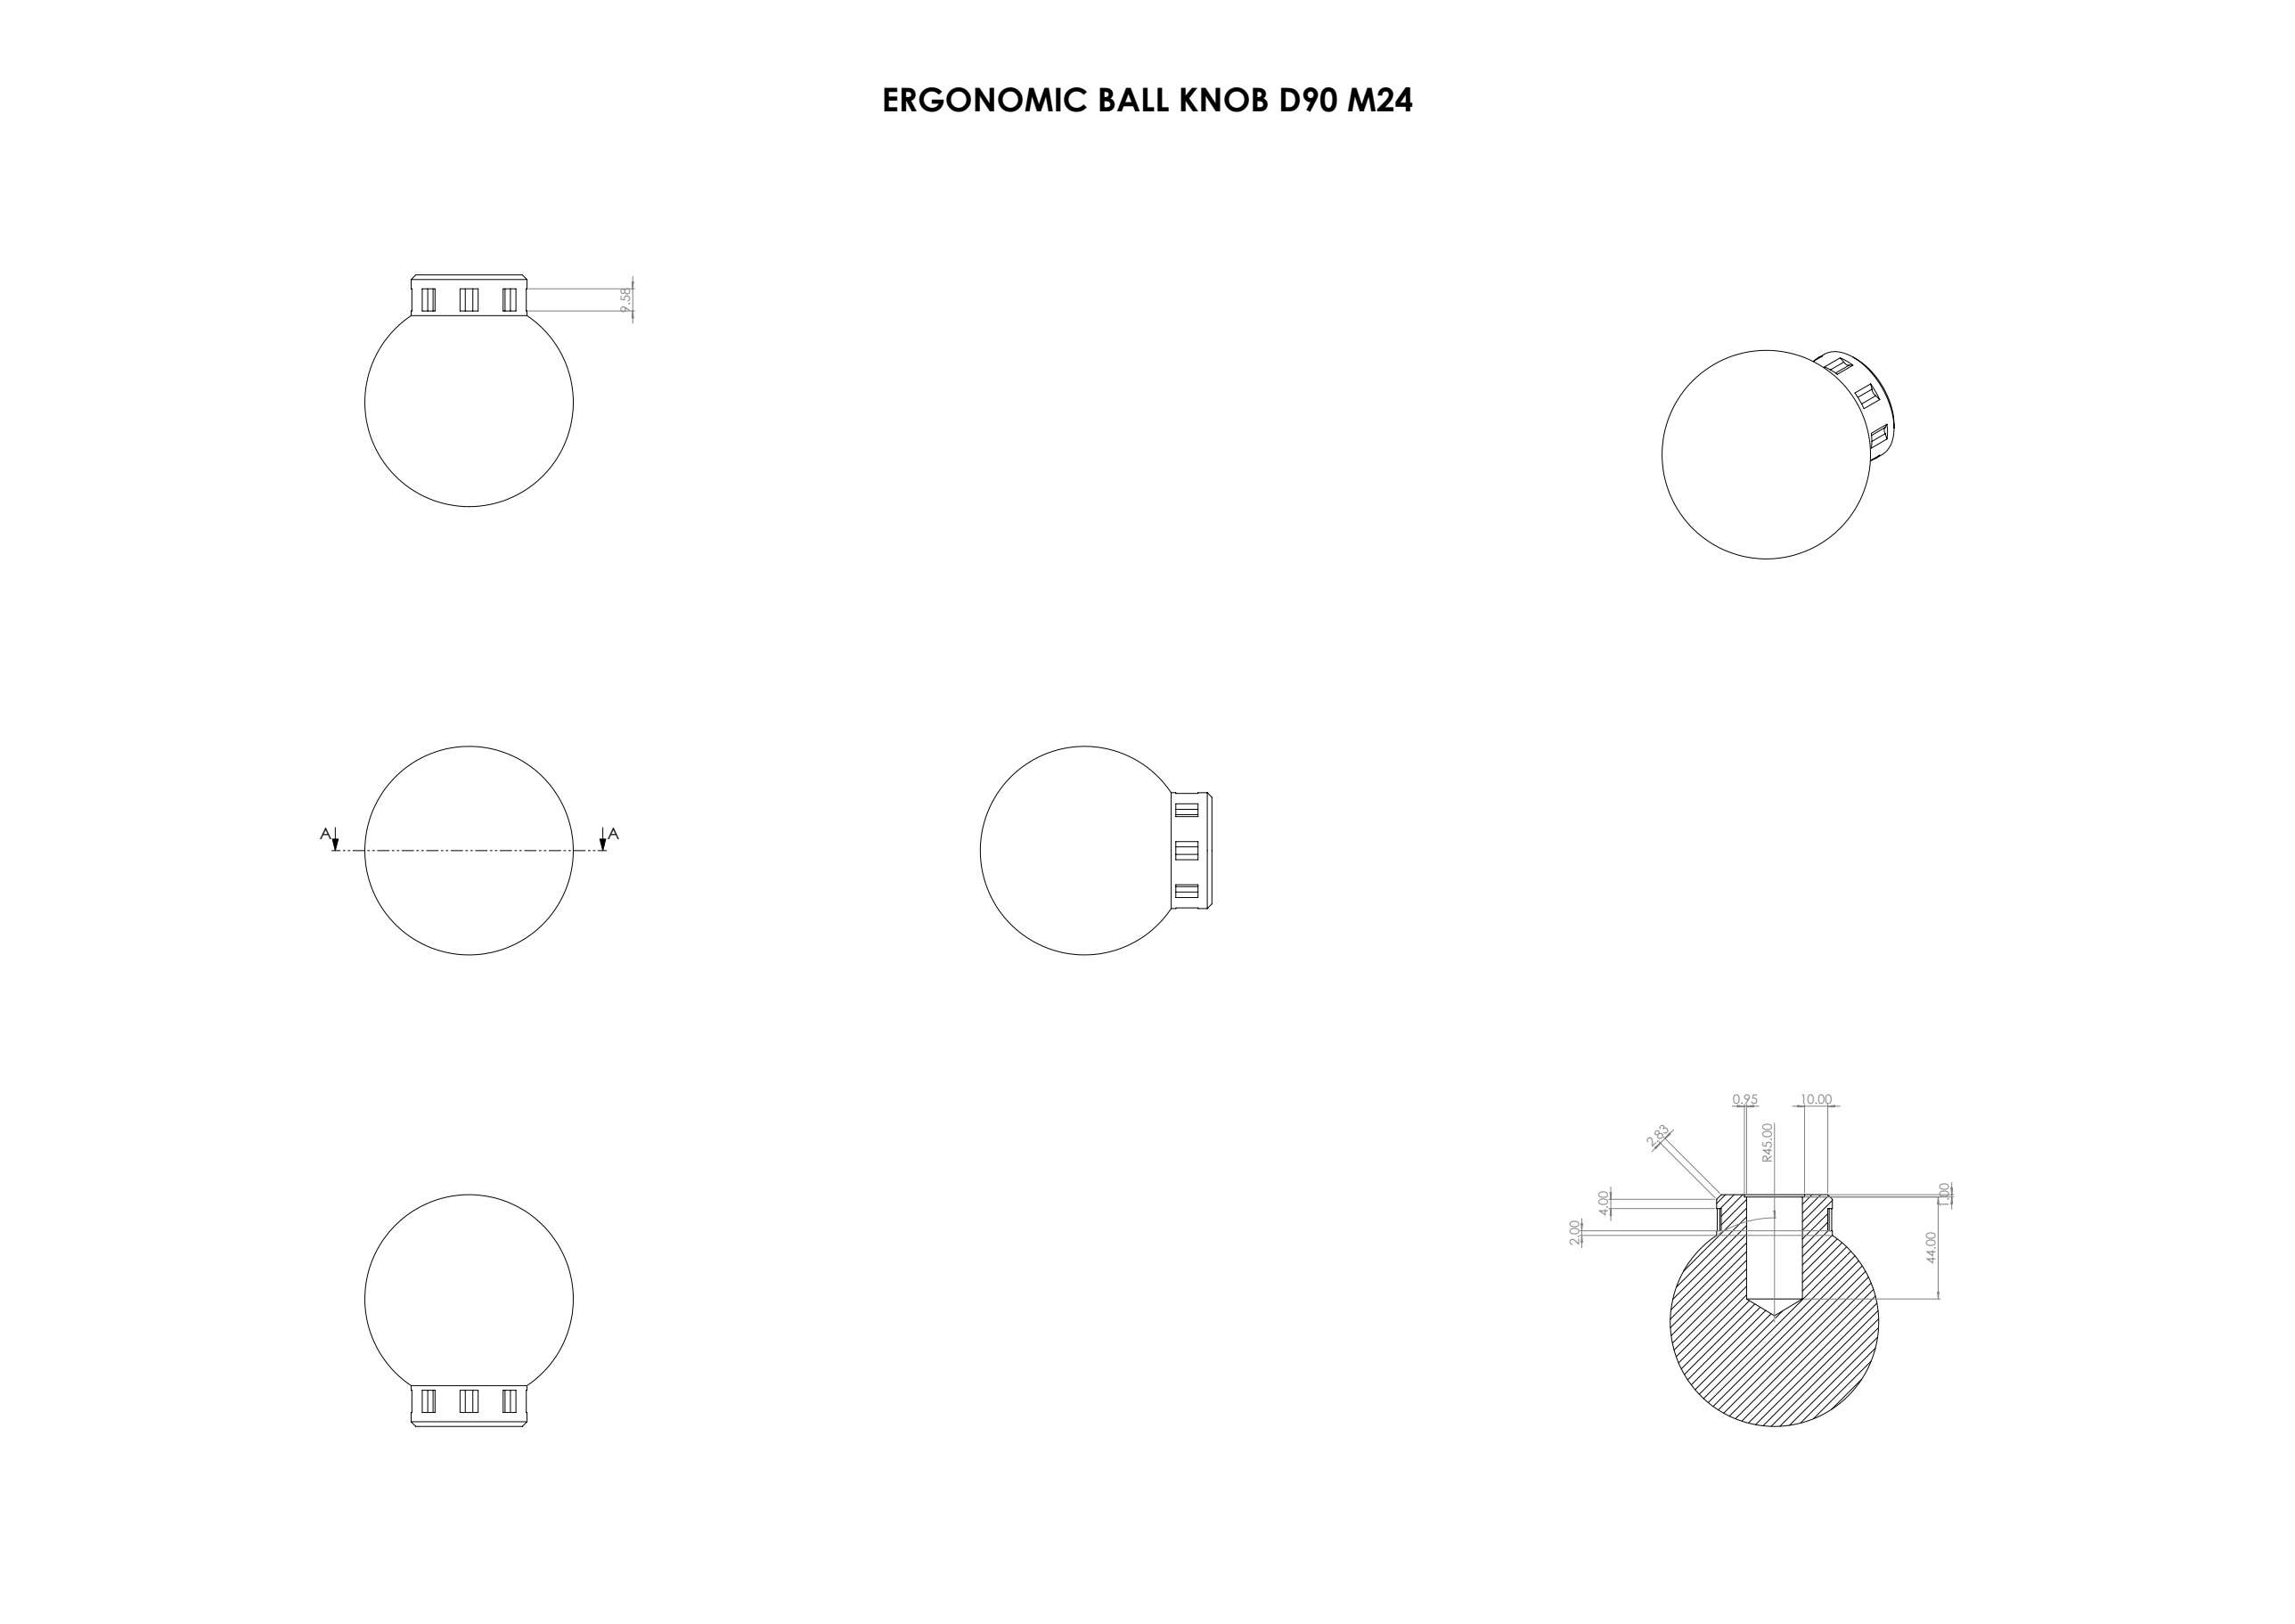
ISO-10303-21;
HEADER;
/* Generated by software containing ST-Developer
 * from STEP Tools, Inc. (www.steptools.com) 
 */

FILE_DESCRIPTION(
/* description */ (''),
/* implementation_level */ '2;1');

FILE_NAME(
/* name */ '06_Ergonomic_Ball_Knob_D90_M24.step',
/* time_stamp */ '2026-10-19T23:58:09-07:00',
/* author */ (''),
/* organization */ (''),
/* preprocessor_version */ 'ST-DEVELOPER v20.2',
/* originating_system */ 'Autodesk Translation Framework v15.15.0.0',
/* authorisation */ '');

FILE_SCHEMA (('AP203_CONFIGURATION_CONTROLLED_3D_DESIGN_OF_MECHANICAL_PARTS_AND_ASSEMBLIES_MIM_LF { 1 0 10303 203 3 1 4 }',
'AUTOMOTIVE_DESIGN { 1 0 10303 214 3 1 1 }','INTEGRATED_CNC_SCHEMA','MODEL_BASED_INTEGRATED_MANUFACTURING_SCHEMA',
'PROCESS_PLANNING_SCHEMA','AP242_MANAGED_MODEL_BASED_3D_ENGINEERING_MIM_LF { 1 0 10303 442 3 1 4 }'));
ENDSEC;

DATA;
#10=MECHANICAL_DESIGN_GEOMETRIC_PRESENTATION_REPRESENTATION('',(#419),#70757);
#135=SPHERICAL_SURFACE('',#28394,4.5);
#389=SHAPE_REPRESENTATION_RELATIONSHIP('SRR','None',#70830,#404);
#404=ADVANCED_BREP_SHAPE_REPRESENTATION('',(#479),#70754);
#419=STYLED_ITEM('',(#71040),#479);
#479=MANIFOLD_SOLID_BREP('Knob',#26884);
#730=CYLINDRICAL_SURFACE('',#28307,0.25);
#731=CYLINDRICAL_SURFACE('',#28312,0.25);
#732=CYLINDRICAL_SURFACE('',#28317,0.25);
#733=CYLINDRICAL_SURFACE('',#28322,0.25);
#734=CYLINDRICAL_SURFACE('',#28327,0.25);
#735=CYLINDRICAL_SURFACE('',#28332,0.25);
#736=CYLINDRICAL_SURFACE('',#28337,0.25);
#737=CYLINDRICAL_SURFACE('',#28342,0.25);
#738=CYLINDRICAL_SURFACE('',#28380,1.3);
#739=CYLINDRICAL_SURFACE('',#28385,1.205);
#740=CYLINDRICAL_SURFACE('',#28392,2.5);
#878=FACE_BOUND('',#5169,.T.);
#879=FACE_BOUND('',#5173,.T.);
#880=FACE_BOUND('',#5176,.T.);
#881=FACE_BOUND('',#5177,.T.);
#882=FACE_BOUND('',#5178,.T.);
#883=FACE_BOUND('',#5179,.T.);
#884=FACE_BOUND('',#5180,.T.);
#885=FACE_BOUND('',#5181,.T.);
#886=FACE_BOUND('',#5182,.T.);
#2392=PLANE('',#28306);
#2393=PLANE('',#28310);
#2394=PLANE('',#28311);
#2395=PLANE('',#28315);
#2396=PLANE('',#28316);
#2397=PLANE('',#28320);
#2398=PLANE('',#28321);
#2399=PLANE('',#28325);
#2400=PLANE('',#28326);
#2401=PLANE('',#28330);
#2402=PLANE('',#28331);
#2403=PLANE('',#28335);
#2404=PLANE('',#28336);
#2405=PLANE('',#28340);
#2406=PLANE('',#28341);
#2407=PLANE('',#28345);
#2408=PLANE('',#28346);
#2409=PLANE('',#28348);
#2410=PLANE('',#28350);
#2411=PLANE('',#28353);
#2412=PLANE('',#28356);
#2413=PLANE('',#28358);
#2414=PLANE('',#28360);
#2415=PLANE('',#28362);
#2416=PLANE('',#28364);
#2417=PLANE('',#28366);
#2418=PLANE('',#28368);
#2419=PLANE('',#28370);
#2420=PLANE('',#28372);
#2421=PLANE('',#28374);
#2422=PLANE('',#28376);
#2423=PLANE('',#28378);
#2424=PLANE('',#28383);
#2425=PLANE('',#28388);
#3605=FACE_OUTER_BOUND('',#5127,.T.);
#3606=FACE_OUTER_BOUND('',#5128,.T.);
#3607=FACE_OUTER_BOUND('',#5129,.T.);
#3608=FACE_OUTER_BOUND('',#5130,.T.);
#3609=FACE_OUTER_BOUND('',#5131,.T.);
#3610=FACE_OUTER_BOUND('',#5132,.T.);
#3611=FACE_OUTER_BOUND('',#5133,.T.);
#3612=FACE_OUTER_BOUND('',#5134,.T.);
#3613=FACE_OUTER_BOUND('',#5135,.T.);
#3614=FACE_OUTER_BOUND('',#5136,.T.);
#3615=FACE_OUTER_BOUND('',#5137,.T.);
#3616=FACE_OUTER_BOUND('',#5138,.T.);
#3617=FACE_OUTER_BOUND('',#5139,.T.);
#3618=FACE_OUTER_BOUND('',#5140,.T.);
#3619=FACE_OUTER_BOUND('',#5141,.T.);
#3620=FACE_OUTER_BOUND('',#5142,.T.);
#3621=FACE_OUTER_BOUND('',#5143,.T.);
#3622=FACE_OUTER_BOUND('',#5144,.T.);
#3623=FACE_OUTER_BOUND('',#5145,.T.);
#3624=FACE_OUTER_BOUND('',#5146,.T.);
#3625=FACE_OUTER_BOUND('',#5147,.T.);
#3626=FACE_OUTER_BOUND('',#5148,.T.);
#3627=FACE_OUTER_BOUND('',#5149,.T.);
#3628=FACE_OUTER_BOUND('',#5150,.T.);
#3629=FACE_OUTER_BOUND('',#5151,.T.);
#3630=FACE_OUTER_BOUND('',#5152,.T.);
#3631=FACE_OUTER_BOUND('',#5153,.T.);
#3632=FACE_OUTER_BOUND('',#5154,.T.);
#3633=FACE_OUTER_BOUND('',#5155,.T.);
#3634=FACE_OUTER_BOUND('',#5156,.T.);
#3635=FACE_OUTER_BOUND('',#5157,.T.);
#3636=FACE_OUTER_BOUND('',#5158,.T.);
#3637=FACE_OUTER_BOUND('',#5159,.T.);
#3638=FACE_OUTER_BOUND('',#5160,.T.);
#3639=FACE_OUTER_BOUND('',#5161,.T.);
#3640=FACE_OUTER_BOUND('',#5162,.T.);
#3641=FACE_OUTER_BOUND('',#5163,.T.);
#3642=FACE_OUTER_BOUND('',#5164,.T.);
#3643=FACE_OUTER_BOUND('',#5165,.T.);
#3644=FACE_OUTER_BOUND('',#5166,.T.);
#3645=FACE_OUTER_BOUND('',#5167,.T.);
#3646=FACE_OUTER_BOUND('',#5168,.T.);
#3647=FACE_OUTER_BOUND('',#5170,.T.);
#3648=FACE_OUTER_BOUND('',#5171,.T.);
#3649=FACE_OUTER_BOUND('',#5172,.T.);
#3650=FACE_OUTER_BOUND('',#5174,.T.);
#3651=FACE_OUTER_BOUND('',#5175,.T.);
#3652=FACE_OUTER_BOUND('',#5183,.T.);
#5127=EDGE_LOOP('',(#22944,#22945,#22946,#22947));
#5128=EDGE_LOOP('',(#22948,#22949,#22950,#22951));
#5129=EDGE_LOOP('',(#22952,#22953,#22954,#22955));
#5130=EDGE_LOOP('',(#22956,#22957,#22958,#22959));
#5131=EDGE_LOOP('',(#22960,#22961,#22962,#22963));
#5132=EDGE_LOOP('',(#22964,#22965,#22966,#22967));
#5133=EDGE_LOOP('',(#22968,#22969,#22970,#22971));
#5134=EDGE_LOOP('',(#22972,#22973,#22974,#22975));
#5135=EDGE_LOOP('',(#22976,#22977,#22978,#22979));
#5136=EDGE_LOOP('',(#22980,#22981,#22982,#22983));
#5137=EDGE_LOOP('',(#22984,#22985,#22986,#22987));
#5138=EDGE_LOOP('',(#22988,#22989,#22990,#22991));
#5139=EDGE_LOOP('',(#22992,#22993,#22994,#22995));
#5140=EDGE_LOOP('',(#22996,#22997,#22998,#22999));
#5141=EDGE_LOOP('',(#23000,#23001,#23002,#23003));
#5142=EDGE_LOOP('',(#23004,#23005,#23006,#23007));
#5143=EDGE_LOOP('',(#23008,#23009,#23010,#23011));
#5144=EDGE_LOOP('',(#23012,#23013,#23014,#23015));
#5145=EDGE_LOOP('',(#23016,#23017,#23018,#23019));
#5146=EDGE_LOOP('',(#23020,#23021,#23022,#23023));
#5147=EDGE_LOOP('',(#23024,#23025,#23026,#23027));
#5148=EDGE_LOOP('',(#23028,#23029,#23030,#23031));
#5149=EDGE_LOOP('',(#23032,#23033,#23034,#23035));
#5150=EDGE_LOOP('',(#23036,#23037,#23038,#23039));
#5151=EDGE_LOOP('',(#23040,#23041,#23042,#23043));
#5152=EDGE_LOOP('',(#23044,#23045,#23046,#23047));
#5153=EDGE_LOOP('',(#23048,#23049,#23050,#23051,#23052));
#5154=EDGE_LOOP('',(#23053,#23054,#23055,#23056,#23057));
#5155=EDGE_LOOP('',(#23058,#23059,#23060,#23061));
#5156=EDGE_LOOP('',(#23062,#23063,#23064,#23065));
#5157=EDGE_LOOP('',(#23066,#23067,#23068,#23069));
#5158=EDGE_LOOP('',(#23070,#23071,#23072,#23073));
#5159=EDGE_LOOP('',(#23074,#23075,#23076,#23077));
#5160=EDGE_LOOP('',(#23078,#23079,#23080,#23081));
#5161=EDGE_LOOP('',(#23082,#23083,#23084,#23085));
#5162=EDGE_LOOP('',(#23086,#23087,#23088,#23089));
#5163=EDGE_LOOP('',(#23090,#23091,#23092,#23093));
#5164=EDGE_LOOP('',(#23094,#23095,#23096,#23097));
#5165=EDGE_LOOP('',(#23098,#23099,#23100,#23101));
#5166=EDGE_LOOP('',(#23102,#23103,#23104,#23105));
#5167=EDGE_LOOP('',(#23106,#23107,#23108,#23109));
#5168=EDGE_LOOP('',(#23110));
#5169=EDGE_LOOP('',(#23111));
#5170=EDGE_LOOP('',(#23112,#23113,#23114,#23115));
#5171=EDGE_LOOP('',(#23116,#23117,#23118));
#5172=EDGE_LOOP('',(#23119));
#5173=EDGE_LOOP('',(#23120));
#5174=EDGE_LOOP('',(#23121,#23122,#23123,#23124));
#5175=EDGE_LOOP('',(#23125,#23126,#23127,#23128,#23129,#23130,#23131,#23132,
#23133,#23134,#23135,#23136));
#5176=EDGE_LOOP('',(#23137,#23138,#23139,#23140));
#5177=EDGE_LOOP('',(#23141,#23142,#23143,#23144));
#5178=EDGE_LOOP('',(#23145,#23146,#23147,#23148));
#5179=EDGE_LOOP('',(#23149,#23150,#23151,#23152));
#5180=EDGE_LOOP('',(#23153,#23154,#23155,#23156));
#5181=EDGE_LOOP('',(#23157,#23158,#23159,#23160));
#5182=EDGE_LOOP('',(#23161,#23162,#23163,#23164));
#5183=EDGE_LOOP('',(#23165,#23166,#23167));
#7543=LINE('',#63698,#10040);
#7544=LINE('',#63700,#10041);
#7545=LINE('',#63702,#10042);
#7546=LINE('',#63703,#10043);
#7547=LINE('',#63708,#10044);
#7548=LINE('',#63712,#10045);
#7549=LINE('',#63714,#10046);
#7550=LINE('',#63715,#10047);
#7551=LINE('',#63719,#10048);
#7552=LINE('',#63721,#10049);
#7553=LINE('',#63723,#10050);
#7554=LINE('',#63724,#10051);
#7555=LINE('',#63729,#10052);
#7556=LINE('',#63733,#10053);
#7557=LINE('',#63735,#10054);
#7558=LINE('',#63736,#10055);
#7559=LINE('',#63740,#10056);
#7560=LINE('',#63742,#10057);
#7561=LINE('',#63744,#10058);
#7562=LINE('',#63745,#10059);
#7563=LINE('',#63750,#10060);
#7564=LINE('',#63754,#10061);
#7565=LINE('',#63756,#10062);
#7566=LINE('',#63757,#10063);
#7567=LINE('',#63761,#10064);
#7568=LINE('',#63763,#10065);
#7569=LINE('',#63765,#10066);
#7570=LINE('',#63766,#10067);
#7571=LINE('',#63771,#10068);
#7572=LINE('',#63775,#10069);
#7573=LINE('',#63777,#10070);
#7574=LINE('',#63778,#10071);
#7575=LINE('',#63782,#10072);
#7576=LINE('',#63784,#10073);
#7577=LINE('',#63786,#10074);
#7578=LINE('',#63787,#10075);
#7579=LINE('',#63792,#10076);
#7580=LINE('',#63796,#10077);
#7581=LINE('',#63798,#10078);
#7582=LINE('',#63799,#10079);
#7583=LINE('',#63803,#10080);
#7584=LINE('',#63805,#10081);
#7585=LINE('',#63807,#10082);
#7586=LINE('',#63808,#10083);
#7587=LINE('',#63813,#10084);
#7588=LINE('',#63817,#10085);
#7589=LINE('',#63819,#10086);
#7590=LINE('',#63820,#10087);
#7591=LINE('',#63824,#10088);
#7592=LINE('',#63826,#10089);
#7593=LINE('',#63828,#10090);
#7594=LINE('',#63829,#10091);
#7595=LINE('',#63834,#10092);
#7596=LINE('',#63838,#10093);
#7597=LINE('',#63840,#10094);
#7598=LINE('',#63841,#10095);
#7599=LINE('',#63845,#10096);
#7600=LINE('',#63847,#10097);
#7601=LINE('',#63849,#10098);
#7602=LINE('',#63850,#10099);
#7603=LINE('',#63855,#10100);
#7604=LINE('',#63859,#10101);
#7605=LINE('',#63861,#10102);
#7606=LINE('',#63862,#10103);
#7607=LINE('',#63903,#10104);
#7608=LINE('',#63910,#10105);
#7609=LINE('',#63914,#10106);
#7610=LINE('',#63921,#10107);
#7611=LINE('',#63925,#10108);
#7612=LINE('',#63926,#10109);
#10040=VECTOR('',#33406,1.);
#10041=VECTOR('',#33407,1.);
#10042=VECTOR('',#33408,1.);
#10043=VECTOR('',#33409,1.);
#10044=VECTOR('',#33414,1.);
#10045=VECTOR('',#33419,1.);
#10046=VECTOR('',#33420,1.);
#10047=VECTOR('',#33421,1.);
#10048=VECTOR('',#33424,1.);
#10049=VECTOR('',#33425,1.);
#10050=VECTOR('',#33426,1.);
#10051=VECTOR('',#33427,1.);
#10052=VECTOR('',#33432,1.);
#10053=VECTOR('',#33437,1.);
#10054=VECTOR('',#33438,1.);
#10055=VECTOR('',#33439,1.);
#10056=VECTOR('',#33442,1.);
#10057=VECTOR('',#33443,1.);
#10058=VECTOR('',#33444,1.);
#10059=VECTOR('',#33445,1.);
#10060=VECTOR('',#33450,1.);
#10061=VECTOR('',#33455,1.);
#10062=VECTOR('',#33456,1.);
#10063=VECTOR('',#33457,1.);
#10064=VECTOR('',#33460,1.);
#10065=VECTOR('',#33461,1.);
#10066=VECTOR('',#33462,1.);
#10067=VECTOR('',#33463,1.);
#10068=VECTOR('',#33468,1.);
#10069=VECTOR('',#33473,1.);
#10070=VECTOR('',#33474,1.);
#10071=VECTOR('',#33475,1.);
#10072=VECTOR('',#33478,1.);
#10073=VECTOR('',#33479,1.);
#10074=VECTOR('',#33480,1.);
#10075=VECTOR('',#33481,1.);
#10076=VECTOR('',#33486,1.);
#10077=VECTOR('',#33491,1.);
#10078=VECTOR('',#33492,1.);
#10079=VECTOR('',#33493,1.);
#10080=VECTOR('',#33496,1.);
#10081=VECTOR('',#33497,1.);
#10082=VECTOR('',#33498,1.);
#10083=VECTOR('',#33499,1.);
#10084=VECTOR('',#33504,1.);
#10085=VECTOR('',#33509,1.);
#10086=VECTOR('',#33510,1.);
#10087=VECTOR('',#33511,1.);
#10088=VECTOR('',#33514,1.);
#10089=VECTOR('',#33515,1.);
#10090=VECTOR('',#33516,1.);
#10091=VECTOR('',#33517,1.);
#10092=VECTOR('',#33522,1.);
#10093=VECTOR('',#33527,1.);
#10094=VECTOR('',#33528,1.);
#10095=VECTOR('',#33529,1.);
#10096=VECTOR('',#33532,1.);
#10097=VECTOR('',#33533,1.);
#10098=VECTOR('',#33534,1.);
#10099=VECTOR('',#33535,1.);
#10100=VECTOR('',#33540,1.);
#10101=VECTOR('',#33545,1.);
#10102=VECTOR('',#33546,1.);
#10103=VECTOR('',#33547,1.);
#10104=VECTOR('',#33620,1.3);
#10105=VECTOR('',#33629,1.205);
#10106=VECTOR('',#33634,1.205);
#10107=VECTOR('',#33643,2.4);
#10108=VECTOR('',#33648,2.5);
#10109=VECTOR('',#33649,2.5);
#10881=CIRCLE('',#28308,0.25);
#10882=CIRCLE('',#28309,0.25);
#10883=CIRCLE('',#28313,0.25);
#10884=CIRCLE('',#28314,0.25);
#10885=CIRCLE('',#28318,0.25);
#10886=CIRCLE('',#28319,0.25);
#10887=CIRCLE('',#28323,0.25);
#10888=CIRCLE('',#28324,0.25);
#10889=CIRCLE('',#28328,0.25);
#10890=CIRCLE('',#28329,0.25);
#10891=CIRCLE('',#28333,0.25);
#10892=CIRCLE('',#28334,0.25);
#10893=CIRCLE('',#28338,0.25);
#10894=CIRCLE('',#28339,0.25);
#10895=CIRCLE('',#28343,0.25);
#10896=CIRCLE('',#28344,0.25);
#10897=CIRCLE('',#28347,2.5);
#10898=CIRCLE('',#28349,2.5);
#10899=CIRCLE('',#28351,2.5);
#10900=CIRCLE('',#28352,2.5);
#10901=CIRCLE('',#28354,2.5);
#10902=CIRCLE('',#28355,2.5);
#10903=CIRCLE('',#28357,2.5);
#10904=CIRCLE('',#28359,2.5);
#10905=CIRCLE('',#28361,2.5);
#10906=CIRCLE('',#28363,2.5);
#10907=CIRCLE('',#28365,2.5);
#10908=CIRCLE('',#28367,2.5);
#10909=CIRCLE('',#28369,2.5);
#10910=CIRCLE('',#28371,2.5);
#10911=CIRCLE('',#28373,2.5);
#10912=CIRCLE('',#28375,2.5);
#10913=CIRCLE('',#28377,2.5);
#10914=CIRCLE('',#28379,2.5);
#10915=CIRCLE('',#28381,1.3);
#10916=CIRCLE('',#28382,1.3);
#10917=CIRCLE('',#28384,1.205);
#10918=CIRCLE('',#28386,1.205);
#10919=CIRCLE('',#28389,2.3);
#10920=CIRCLE('',#28391,2.5);
#10921=CIRCLE('',#28393,2.5);
#10922=CIRCLE('',#28395,4.5);
#12856=VERTEX_POINT('',#63696);
#12857=VERTEX_POINT('',#63697);
#12858=VERTEX_POINT('',#63699);
#12859=VERTEX_POINT('',#63701);
#12860=VERTEX_POINT('',#63705);
#12861=VERTEX_POINT('',#63707);
#12862=VERTEX_POINT('',#63711);
#12863=VERTEX_POINT('',#63713);
#12864=VERTEX_POINT('',#63717);
#12865=VERTEX_POINT('',#63718);
#12866=VERTEX_POINT('',#63720);
#12867=VERTEX_POINT('',#63722);
#12868=VERTEX_POINT('',#63726);
#12869=VERTEX_POINT('',#63728);
#12870=VERTEX_POINT('',#63732);
#12871=VERTEX_POINT('',#63734);
#12872=VERTEX_POINT('',#63738);
#12873=VERTEX_POINT('',#63739);
#12874=VERTEX_POINT('',#63741);
#12875=VERTEX_POINT('',#63743);
#12876=VERTEX_POINT('',#63747);
#12877=VERTEX_POINT('',#63749);
#12878=VERTEX_POINT('',#63753);
#12879=VERTEX_POINT('',#63755);
#12880=VERTEX_POINT('',#63759);
#12881=VERTEX_POINT('',#63760);
#12882=VERTEX_POINT('',#63762);
#12883=VERTEX_POINT('',#63764);
#12884=VERTEX_POINT('',#63768);
#12885=VERTEX_POINT('',#63770);
#12886=VERTEX_POINT('',#63774);
#12887=VERTEX_POINT('',#63776);
#12888=VERTEX_POINT('',#63780);
#12889=VERTEX_POINT('',#63781);
#12890=VERTEX_POINT('',#63783);
#12891=VERTEX_POINT('',#63785);
#12892=VERTEX_POINT('',#63789);
#12893=VERTEX_POINT('',#63791);
#12894=VERTEX_POINT('',#63795);
#12895=VERTEX_POINT('',#63797);
#12896=VERTEX_POINT('',#63801);
#12897=VERTEX_POINT('',#63802);
#12898=VERTEX_POINT('',#63804);
#12899=VERTEX_POINT('',#63806);
#12900=VERTEX_POINT('',#63810);
#12901=VERTEX_POINT('',#63812);
#12902=VERTEX_POINT('',#63816);
#12903=VERTEX_POINT('',#63818);
#12904=VERTEX_POINT('',#63822);
#12905=VERTEX_POINT('',#63823);
#12906=VERTEX_POINT('',#63825);
#12907=VERTEX_POINT('',#63827);
#12908=VERTEX_POINT('',#63831);
#12909=VERTEX_POINT('',#63833);
#12910=VERTEX_POINT('',#63837);
#12911=VERTEX_POINT('',#63839);
#12912=VERTEX_POINT('',#63843);
#12913=VERTEX_POINT('',#63844);
#12914=VERTEX_POINT('',#63846);
#12915=VERTEX_POINT('',#63848);
#12916=VERTEX_POINT('',#63852);
#12917=VERTEX_POINT('',#63854);
#12918=VERTEX_POINT('',#63858);
#12919=VERTEX_POINT('',#63860);
#12920=VERTEX_POINT('',#63868);
#12921=VERTEX_POINT('',#63872);
#12922=VERTEX_POINT('',#63900);
#12923=VERTEX_POINT('',#63902);
#12924=VERTEX_POINT('',#63906);
#12925=VERTEX_POINT('',#63909);
#12926=VERTEX_POINT('',#63913);
#12927=VERTEX_POINT('',#63916);
#12928=VERTEX_POINT('',#63919);
#12929=VERTEX_POINT('',#63923);
#12930=VERTEX_POINT('',#63928);
#16325=EDGE_CURVE('',#12856,#12857,#7543,.F.);
#16326=EDGE_CURVE('',#12857,#12858,#7544,.T.);
#16327=EDGE_CURVE('',#12858,#12859,#7545,.F.);
#16328=EDGE_CURVE('',#12859,#12856,#7546,.T.);
#16329=EDGE_CURVE('',#12860,#12857,#10881,.T.);
#16330=EDGE_CURVE('',#12861,#12860,#7547,.T.);
#16331=EDGE_CURVE('',#12861,#12858,#10882,.T.);
#16332=EDGE_CURVE('',#12862,#12861,#7548,.F.);
#16333=EDGE_CURVE('',#12860,#12863,#7549,.F.);
#16334=EDGE_CURVE('',#12863,#12862,#7550,.T.);
#16335=EDGE_CURVE('',#12864,#12865,#7551,.F.);
#16336=EDGE_CURVE('',#12865,#12866,#7552,.T.);
#16337=EDGE_CURVE('',#12866,#12867,#7553,.F.);
#16338=EDGE_CURVE('',#12867,#12864,#7554,.T.);
#16339=EDGE_CURVE('',#12865,#12868,#10883,.T.);
#16340=EDGE_CURVE('',#12869,#12868,#7555,.T.);
#16341=EDGE_CURVE('',#12866,#12869,#10884,.T.);
#16342=EDGE_CURVE('',#12870,#12869,#7556,.F.);
#16343=EDGE_CURVE('',#12868,#12871,#7557,.F.);
#16344=EDGE_CURVE('',#12871,#12870,#7558,.T.);
#16345=EDGE_CURVE('',#12872,#12873,#7559,.F.);
#16346=EDGE_CURVE('',#12873,#12874,#7560,.T.);
#16347=EDGE_CURVE('',#12874,#12875,#7561,.F.);
#16348=EDGE_CURVE('',#12875,#12872,#7562,.T.);
#16349=EDGE_CURVE('',#12876,#12873,#10885,.T.);
#16350=EDGE_CURVE('',#12877,#12876,#7563,.T.);
#16351=EDGE_CURVE('',#12877,#12874,#10886,.T.);
#16352=EDGE_CURVE('',#12878,#12877,#7564,.F.);
#16353=EDGE_CURVE('',#12876,#12879,#7565,.F.);
#16354=EDGE_CURVE('',#12879,#12878,#7566,.T.);
#16355=EDGE_CURVE('',#12880,#12881,#7567,.F.);
#16356=EDGE_CURVE('',#12881,#12882,#7568,.T.);
#16357=EDGE_CURVE('',#12882,#12883,#7569,.F.);
#16358=EDGE_CURVE('',#12883,#12880,#7570,.T.);
#16359=EDGE_CURVE('',#12881,#12884,#10887,.T.);
#16360=EDGE_CURVE('',#12885,#12884,#7571,.T.);
#16361=EDGE_CURVE('',#12882,#12885,#10888,.T.);
#16362=EDGE_CURVE('',#12886,#12885,#7572,.F.);
#16363=EDGE_CURVE('',#12884,#12887,#7573,.F.);
#16364=EDGE_CURVE('',#12887,#12886,#7574,.T.);
#16365=EDGE_CURVE('',#12888,#12889,#7575,.F.);
#16366=EDGE_CURVE('',#12889,#12890,#7576,.T.);
#16367=EDGE_CURVE('',#12890,#12891,#7577,.F.);
#16368=EDGE_CURVE('',#12891,#12888,#7578,.T.);
#16369=EDGE_CURVE('',#12892,#12889,#10889,.T.);
#16370=EDGE_CURVE('',#12893,#12892,#7579,.T.);
#16371=EDGE_CURVE('',#12893,#12890,#10890,.T.);
#16372=EDGE_CURVE('',#12894,#12893,#7580,.F.);
#16373=EDGE_CURVE('',#12892,#12895,#7581,.F.);
#16374=EDGE_CURVE('',#12895,#12894,#7582,.T.);
#16375=EDGE_CURVE('',#12896,#12897,#7583,.F.);
#16376=EDGE_CURVE('',#12897,#12898,#7584,.T.);
#16377=EDGE_CURVE('',#12898,#12899,#7585,.F.);
#16378=EDGE_CURVE('',#12899,#12896,#7586,.T.);
#16379=EDGE_CURVE('',#12897,#12900,#10891,.T.);
#16380=EDGE_CURVE('',#12901,#12900,#7587,.T.);
#16381=EDGE_CURVE('',#12898,#12901,#10892,.T.);
#16382=EDGE_CURVE('',#12902,#12901,#7588,.F.);
#16383=EDGE_CURVE('',#12900,#12903,#7589,.F.);
#16384=EDGE_CURVE('',#12903,#12902,#7590,.T.);
#16385=EDGE_CURVE('',#12904,#12905,#7591,.F.);
#16386=EDGE_CURVE('',#12905,#12906,#7592,.T.);
#16387=EDGE_CURVE('',#12906,#12907,#7593,.F.);
#16388=EDGE_CURVE('',#12907,#12904,#7594,.T.);
#16389=EDGE_CURVE('',#12905,#12908,#10893,.T.);
#16390=EDGE_CURVE('',#12909,#12908,#7595,.T.);
#16391=EDGE_CURVE('',#12906,#12909,#10894,.T.);
#16392=EDGE_CURVE('',#12910,#12909,#7596,.F.);
#16393=EDGE_CURVE('',#12908,#12911,#7597,.F.);
#16394=EDGE_CURVE('',#12911,#12910,#7598,.T.);
#16395=EDGE_CURVE('',#12912,#12913,#7599,.F.);
#16396=EDGE_CURVE('',#12913,#12914,#7600,.T.);
#16397=EDGE_CURVE('',#12914,#12915,#7601,.F.);
#16398=EDGE_CURVE('',#12915,#12912,#7602,.T.);
#16399=EDGE_CURVE('',#12913,#12916,#10895,.T.);
#16400=EDGE_CURVE('',#12917,#12916,#7603,.T.);
#16401=EDGE_CURVE('',#12914,#12917,#10896,.T.);
#16402=EDGE_CURVE('',#12918,#12917,#7604,.F.);
#16403=EDGE_CURVE('',#12916,#12919,#7605,.F.);
#16404=EDGE_CURVE('',#12919,#12918,#7606,.T.);
#16405=EDGE_CURVE('',#12919,#12912,#10897,.T.);
#16406=EDGE_CURVE('',#12915,#12918,#10898,.T.);
#16407=EDGE_CURVE('',#12911,#12920,#10899,.T.);
#16408=EDGE_CURVE('',#12920,#12904,#10900,.T.);
#16409=EDGE_CURVE('',#12907,#12921,#10901,.T.);
#16410=EDGE_CURVE('',#12921,#12910,#10902,.T.);
#16411=EDGE_CURVE('',#12903,#12896,#10903,.T.);
#16412=EDGE_CURVE('',#12899,#12902,#10904,.T.);
#16413=EDGE_CURVE('',#12895,#12888,#10905,.T.);
#16414=EDGE_CURVE('',#12891,#12894,#10906,.T.);
#16415=EDGE_CURVE('',#12887,#12880,#10907,.T.);
#16416=EDGE_CURVE('',#12883,#12886,#10908,.T.);
#16417=EDGE_CURVE('',#12879,#12872,#10909,.T.);
#16418=EDGE_CURVE('',#12875,#12878,#10910,.T.);
#16419=EDGE_CURVE('',#12871,#12864,#10911,.T.);
#16420=EDGE_CURVE('',#12867,#12870,#10912,.T.);
#16421=EDGE_CURVE('',#12863,#12856,#10913,.T.);
#16422=EDGE_CURVE('',#12859,#12862,#10914,.T.);
#16423=EDGE_CURVE('',#12922,#12922,#10915,.T.);
#16424=EDGE_CURVE('',#12922,#12923,#7607,.T.);
#16425=EDGE_CURVE('',#12923,#12923,#10916,.T.);
#16426=EDGE_CURVE('',#12924,#12924,#10917,.T.);
#16427=EDGE_CURVE('',#12924,#12925,#7608,.T.);
#16428=EDGE_CURVE('',#12925,#12925,#10918,.T.);
#16429=EDGE_CURVE('',#12925,#12926,#7609,.T.);
#16430=EDGE_CURVE('',#12927,#12927,#10919,.T.);
#16431=EDGE_CURVE('',#12928,#12928,#10920,.T.);
#16432=EDGE_CURVE('',#12928,#12927,#7610,.T.);
#16433=EDGE_CURVE('',#12929,#12929,#10921,.T.);
#16434=EDGE_CURVE('',#12929,#12920,#7611,.T.);
#16435=EDGE_CURVE('',#12921,#12928,#7612,.T.);
#16436=EDGE_CURVE('',#12930,#12929,#10922,.T.);
#22944=ORIENTED_EDGE('',*,*,#16325,.T.);
#22945=ORIENTED_EDGE('',*,*,#16326,.T.);
#22946=ORIENTED_EDGE('',*,*,#16327,.T.);
#22947=ORIENTED_EDGE('',*,*,#16328,.T.);
#22948=ORIENTED_EDGE('',*,*,#16326,.F.);
#22949=ORIENTED_EDGE('',*,*,#16329,.F.);
#22950=ORIENTED_EDGE('',*,*,#16330,.F.);
#22951=ORIENTED_EDGE('',*,*,#16331,.T.);
#22952=ORIENTED_EDGE('',*,*,#16332,.T.);
#22953=ORIENTED_EDGE('',*,*,#16330,.T.);
#22954=ORIENTED_EDGE('',*,*,#16333,.T.);
#22955=ORIENTED_EDGE('',*,*,#16334,.T.);
#22956=ORIENTED_EDGE('',*,*,#16335,.T.);
#22957=ORIENTED_EDGE('',*,*,#16336,.T.);
#22958=ORIENTED_EDGE('',*,*,#16337,.T.);
#22959=ORIENTED_EDGE('',*,*,#16338,.T.);
#22960=ORIENTED_EDGE('',*,*,#16336,.F.);
#22961=ORIENTED_EDGE('',*,*,#16339,.T.);
#22962=ORIENTED_EDGE('',*,*,#16340,.F.);
#22963=ORIENTED_EDGE('',*,*,#16341,.F.);
#22964=ORIENTED_EDGE('',*,*,#16342,.T.);
#22965=ORIENTED_EDGE('',*,*,#16340,.T.);
#22966=ORIENTED_EDGE('',*,*,#16343,.T.);
#22967=ORIENTED_EDGE('',*,*,#16344,.T.);
#22968=ORIENTED_EDGE('',*,*,#16345,.T.);
#22969=ORIENTED_EDGE('',*,*,#16346,.T.);
#22970=ORIENTED_EDGE('',*,*,#16347,.T.);
#22971=ORIENTED_EDGE('',*,*,#16348,.T.);
#22972=ORIENTED_EDGE('',*,*,#16346,.F.);
#22973=ORIENTED_EDGE('',*,*,#16349,.F.);
#22974=ORIENTED_EDGE('',*,*,#16350,.F.);
#22975=ORIENTED_EDGE('',*,*,#16351,.T.);
#22976=ORIENTED_EDGE('',*,*,#16352,.T.);
#22977=ORIENTED_EDGE('',*,*,#16350,.T.);
#22978=ORIENTED_EDGE('',*,*,#16353,.T.);
#22979=ORIENTED_EDGE('',*,*,#16354,.T.);
#22980=ORIENTED_EDGE('',*,*,#16355,.T.);
#22981=ORIENTED_EDGE('',*,*,#16356,.T.);
#22982=ORIENTED_EDGE('',*,*,#16357,.T.);
#22983=ORIENTED_EDGE('',*,*,#16358,.T.);
#22984=ORIENTED_EDGE('',*,*,#16356,.F.);
#22985=ORIENTED_EDGE('',*,*,#16359,.T.);
#22986=ORIENTED_EDGE('',*,*,#16360,.F.);
#22987=ORIENTED_EDGE('',*,*,#16361,.F.);
#22988=ORIENTED_EDGE('',*,*,#16362,.T.);
#22989=ORIENTED_EDGE('',*,*,#16360,.T.);
#22990=ORIENTED_EDGE('',*,*,#16363,.T.);
#22991=ORIENTED_EDGE('',*,*,#16364,.T.);
#22992=ORIENTED_EDGE('',*,*,#16365,.T.);
#22993=ORIENTED_EDGE('',*,*,#16366,.T.);
#22994=ORIENTED_EDGE('',*,*,#16367,.T.);
#22995=ORIENTED_EDGE('',*,*,#16368,.T.);
#22996=ORIENTED_EDGE('',*,*,#16366,.F.);
#22997=ORIENTED_EDGE('',*,*,#16369,.F.);
#22998=ORIENTED_EDGE('',*,*,#16370,.F.);
#22999=ORIENTED_EDGE('',*,*,#16371,.T.);
#23000=ORIENTED_EDGE('',*,*,#16372,.T.);
#23001=ORIENTED_EDGE('',*,*,#16370,.T.);
#23002=ORIENTED_EDGE('',*,*,#16373,.T.);
#23003=ORIENTED_EDGE('',*,*,#16374,.T.);
#23004=ORIENTED_EDGE('',*,*,#16375,.T.);
#23005=ORIENTED_EDGE('',*,*,#16376,.T.);
#23006=ORIENTED_EDGE('',*,*,#16377,.T.);
#23007=ORIENTED_EDGE('',*,*,#16378,.T.);
#23008=ORIENTED_EDGE('',*,*,#16376,.F.);
#23009=ORIENTED_EDGE('',*,*,#16379,.T.);
#23010=ORIENTED_EDGE('',*,*,#16380,.F.);
#23011=ORIENTED_EDGE('',*,*,#16381,.F.);
#23012=ORIENTED_EDGE('',*,*,#16382,.T.);
#23013=ORIENTED_EDGE('',*,*,#16380,.T.);
#23014=ORIENTED_EDGE('',*,*,#16383,.T.);
#23015=ORIENTED_EDGE('',*,*,#16384,.T.);
#23016=ORIENTED_EDGE('',*,*,#16385,.T.);
#23017=ORIENTED_EDGE('',*,*,#16386,.T.);
#23018=ORIENTED_EDGE('',*,*,#16387,.T.);
#23019=ORIENTED_EDGE('',*,*,#16388,.T.);
#23020=ORIENTED_EDGE('',*,*,#16386,.F.);
#23021=ORIENTED_EDGE('',*,*,#16389,.T.);
#23022=ORIENTED_EDGE('',*,*,#16390,.F.);
#23023=ORIENTED_EDGE('',*,*,#16391,.F.);
#23024=ORIENTED_EDGE('',*,*,#16392,.T.);
#23025=ORIENTED_EDGE('',*,*,#16390,.T.);
#23026=ORIENTED_EDGE('',*,*,#16393,.T.);
#23027=ORIENTED_EDGE('',*,*,#16394,.T.);
#23028=ORIENTED_EDGE('',*,*,#16395,.T.);
#23029=ORIENTED_EDGE('',*,*,#16396,.T.);
#23030=ORIENTED_EDGE('',*,*,#16397,.T.);
#23031=ORIENTED_EDGE('',*,*,#16398,.T.);
#23032=ORIENTED_EDGE('',*,*,#16396,.F.);
#23033=ORIENTED_EDGE('',*,*,#16399,.T.);
#23034=ORIENTED_EDGE('',*,*,#16400,.F.);
#23035=ORIENTED_EDGE('',*,*,#16401,.F.);
#23036=ORIENTED_EDGE('',*,*,#16402,.T.);
#23037=ORIENTED_EDGE('',*,*,#16400,.T.);
#23038=ORIENTED_EDGE('',*,*,#16403,.T.);
#23039=ORIENTED_EDGE('',*,*,#16404,.T.);
#23040=ORIENTED_EDGE('',*,*,#16405,.F.);
#23041=ORIENTED_EDGE('',*,*,#16403,.F.);
#23042=ORIENTED_EDGE('',*,*,#16399,.F.);
#23043=ORIENTED_EDGE('',*,*,#16395,.F.);
#23044=ORIENTED_EDGE('',*,*,#16406,.F.);
#23045=ORIENTED_EDGE('',*,*,#16397,.F.);
#23046=ORIENTED_EDGE('',*,*,#16401,.T.);
#23047=ORIENTED_EDGE('',*,*,#16402,.F.);
#23048=ORIENTED_EDGE('',*,*,#16407,.F.);
#23049=ORIENTED_EDGE('',*,*,#16393,.F.);
#23050=ORIENTED_EDGE('',*,*,#16389,.F.);
#23051=ORIENTED_EDGE('',*,*,#16385,.F.);
#23052=ORIENTED_EDGE('',*,*,#16408,.F.);
#23053=ORIENTED_EDGE('',*,*,#16409,.F.);
#23054=ORIENTED_EDGE('',*,*,#16387,.F.);
#23055=ORIENTED_EDGE('',*,*,#16391,.T.);
#23056=ORIENTED_EDGE('',*,*,#16392,.F.);
#23057=ORIENTED_EDGE('',*,*,#16410,.F.);
#23058=ORIENTED_EDGE('',*,*,#16411,.F.);
#23059=ORIENTED_EDGE('',*,*,#16383,.F.);
#23060=ORIENTED_EDGE('',*,*,#16379,.F.);
#23061=ORIENTED_EDGE('',*,*,#16375,.F.);
#23062=ORIENTED_EDGE('',*,*,#16412,.F.);
#23063=ORIENTED_EDGE('',*,*,#16377,.F.);
#23064=ORIENTED_EDGE('',*,*,#16381,.T.);
#23065=ORIENTED_EDGE('',*,*,#16382,.F.);
#23066=ORIENTED_EDGE('',*,*,#16413,.F.);
#23067=ORIENTED_EDGE('',*,*,#16373,.F.);
#23068=ORIENTED_EDGE('',*,*,#16369,.T.);
#23069=ORIENTED_EDGE('',*,*,#16365,.F.);
#23070=ORIENTED_EDGE('',*,*,#16414,.F.);
#23071=ORIENTED_EDGE('',*,*,#16367,.F.);
#23072=ORIENTED_EDGE('',*,*,#16371,.F.);
#23073=ORIENTED_EDGE('',*,*,#16372,.F.);
#23074=ORIENTED_EDGE('',*,*,#16415,.F.);
#23075=ORIENTED_EDGE('',*,*,#16363,.F.);
#23076=ORIENTED_EDGE('',*,*,#16359,.F.);
#23077=ORIENTED_EDGE('',*,*,#16355,.F.);
#23078=ORIENTED_EDGE('',*,*,#16416,.F.);
#23079=ORIENTED_EDGE('',*,*,#16357,.F.);
#23080=ORIENTED_EDGE('',*,*,#16361,.T.);
#23081=ORIENTED_EDGE('',*,*,#16362,.F.);
#23082=ORIENTED_EDGE('',*,*,#16417,.F.);
#23083=ORIENTED_EDGE('',*,*,#16353,.F.);
#23084=ORIENTED_EDGE('',*,*,#16349,.T.);
#23085=ORIENTED_EDGE('',*,*,#16345,.F.);
#23086=ORIENTED_EDGE('',*,*,#16418,.F.);
#23087=ORIENTED_EDGE('',*,*,#16347,.F.);
#23088=ORIENTED_EDGE('',*,*,#16351,.F.);
#23089=ORIENTED_EDGE('',*,*,#16352,.F.);
#23090=ORIENTED_EDGE('',*,*,#16419,.F.);
#23091=ORIENTED_EDGE('',*,*,#16343,.F.);
#23092=ORIENTED_EDGE('',*,*,#16339,.F.);
#23093=ORIENTED_EDGE('',*,*,#16335,.F.);
#23094=ORIENTED_EDGE('',*,*,#16420,.F.);
#23095=ORIENTED_EDGE('',*,*,#16337,.F.);
#23096=ORIENTED_EDGE('',*,*,#16341,.T.);
#23097=ORIENTED_EDGE('',*,*,#16342,.F.);
#23098=ORIENTED_EDGE('',*,*,#16421,.F.);
#23099=ORIENTED_EDGE('',*,*,#16333,.F.);
#23100=ORIENTED_EDGE('',*,*,#16329,.T.);
#23101=ORIENTED_EDGE('',*,*,#16325,.F.);
#23102=ORIENTED_EDGE('',*,*,#16422,.F.);
#23103=ORIENTED_EDGE('',*,*,#16327,.F.);
#23104=ORIENTED_EDGE('',*,*,#16331,.F.);
#23105=ORIENTED_EDGE('',*,*,#16332,.F.);
#23106=ORIENTED_EDGE('',*,*,#16423,.F.);
#23107=ORIENTED_EDGE('',*,*,#16424,.T.);
#23108=ORIENTED_EDGE('',*,*,#16425,.T.);
#23109=ORIENTED_EDGE('',*,*,#16424,.F.);
#23110=ORIENTED_EDGE('',*,*,#16425,.F.);
#23111=ORIENTED_EDGE('',*,*,#16426,.T.);
#23112=ORIENTED_EDGE('',*,*,#16426,.F.);
#23113=ORIENTED_EDGE('',*,*,#16427,.T.);
#23114=ORIENTED_EDGE('',*,*,#16428,.T.);
#23115=ORIENTED_EDGE('',*,*,#16427,.F.);
#23116=ORIENTED_EDGE('',*,*,#16428,.F.);
#23117=ORIENTED_EDGE('',*,*,#16429,.T.);
#23118=ORIENTED_EDGE('',*,*,#16429,.F.);
#23119=ORIENTED_EDGE('',*,*,#16430,.F.);
#23120=ORIENTED_EDGE('',*,*,#16423,.T.);
#23121=ORIENTED_EDGE('',*,*,#16431,.F.);
#23122=ORIENTED_EDGE('',*,*,#16432,.T.);
#23123=ORIENTED_EDGE('',*,*,#16430,.T.);
#23124=ORIENTED_EDGE('',*,*,#16432,.F.);
#23125=ORIENTED_EDGE('',*,*,#16433,.F.);
#23126=ORIENTED_EDGE('',*,*,#16434,.T.);
#23127=ORIENTED_EDGE('',*,*,#16408,.T.);
#23128=ORIENTED_EDGE('',*,*,#16388,.F.);
#23129=ORIENTED_EDGE('',*,*,#16409,.T.);
#23130=ORIENTED_EDGE('',*,*,#16435,.T.);
#23131=ORIENTED_EDGE('',*,*,#16431,.T.);
#23132=ORIENTED_EDGE('',*,*,#16435,.F.);
#23133=ORIENTED_EDGE('',*,*,#16410,.T.);
#23134=ORIENTED_EDGE('',*,*,#16394,.F.);
#23135=ORIENTED_EDGE('',*,*,#16407,.T.);
#23136=ORIENTED_EDGE('',*,*,#16434,.F.);
#23137=ORIENTED_EDGE('',*,*,#16422,.T.);
#23138=ORIENTED_EDGE('',*,*,#16334,.F.);
#23139=ORIENTED_EDGE('',*,*,#16421,.T.);
#23140=ORIENTED_EDGE('',*,*,#16328,.F.);
#23141=ORIENTED_EDGE('',*,*,#16420,.T.);
#23142=ORIENTED_EDGE('',*,*,#16344,.F.);
#23143=ORIENTED_EDGE('',*,*,#16419,.T.);
#23144=ORIENTED_EDGE('',*,*,#16338,.F.);
#23145=ORIENTED_EDGE('',*,*,#16418,.T.);
#23146=ORIENTED_EDGE('',*,*,#16354,.F.);
#23147=ORIENTED_EDGE('',*,*,#16417,.T.);
#23148=ORIENTED_EDGE('',*,*,#16348,.F.);
#23149=ORIENTED_EDGE('',*,*,#16416,.T.);
#23150=ORIENTED_EDGE('',*,*,#16364,.F.);
#23151=ORIENTED_EDGE('',*,*,#16415,.T.);
#23152=ORIENTED_EDGE('',*,*,#16358,.F.);
#23153=ORIENTED_EDGE('',*,*,#16414,.T.);
#23154=ORIENTED_EDGE('',*,*,#16374,.F.);
#23155=ORIENTED_EDGE('',*,*,#16413,.T.);
#23156=ORIENTED_EDGE('',*,*,#16368,.F.);
#23157=ORIENTED_EDGE('',*,*,#16412,.T.);
#23158=ORIENTED_EDGE('',*,*,#16384,.F.);
#23159=ORIENTED_EDGE('',*,*,#16411,.T.);
#23160=ORIENTED_EDGE('',*,*,#16378,.F.);
#23161=ORIENTED_EDGE('',*,*,#16406,.T.);
#23162=ORIENTED_EDGE('',*,*,#16404,.F.);
#23163=ORIENTED_EDGE('',*,*,#16405,.T.);
#23164=ORIENTED_EDGE('',*,*,#16398,.F.);
#23165=ORIENTED_EDGE('',*,*,#16433,.T.);
#23166=ORIENTED_EDGE('',*,*,#16436,.F.);
#23167=ORIENTED_EDGE('',*,*,#16436,.T.);
#25347=CONICAL_SURFACE('',#28387,1.205,1.02974425867666);
#25348=CONICAL_SURFACE('',#28390,2.4,0.785398163397442);
#26418=ADVANCED_FACE('',(#3605),#2392,.T.);
#26419=ADVANCED_FACE('',(#3606),#730,.F.);
#26420=ADVANCED_FACE('',(#3607),#2393,.T.);
#26421=ADVANCED_FACE('',(#3608),#2394,.T.);
#26422=ADVANCED_FACE('',(#3609),#731,.F.);
#26423=ADVANCED_FACE('',(#3610),#2395,.T.);
#26424=ADVANCED_FACE('',(#3611),#2396,.T.);
#26425=ADVANCED_FACE('',(#3612),#732,.F.);
#26426=ADVANCED_FACE('',(#3613),#2397,.T.);
#26427=ADVANCED_FACE('',(#3614),#2398,.T.);
#26428=ADVANCED_FACE('',(#3615),#733,.F.);
#26429=ADVANCED_FACE('',(#3616),#2399,.T.);
#26430=ADVANCED_FACE('',(#3617),#2400,.T.);
#26431=ADVANCED_FACE('',(#3618),#734,.F.);
#26432=ADVANCED_FACE('',(#3619),#2401,.T.);
#26433=ADVANCED_FACE('',(#3620),#2402,.T.);
#26434=ADVANCED_FACE('',(#3621),#735,.F.);
#26435=ADVANCED_FACE('',(#3622),#2403,.T.);
#26436=ADVANCED_FACE('',(#3623),#2404,.T.);
#26437=ADVANCED_FACE('',(#3624),#736,.F.);
#26438=ADVANCED_FACE('',(#3625),#2405,.T.);
#26439=ADVANCED_FACE('',(#3626),#2406,.T.);
#26440=ADVANCED_FACE('',(#3627),#737,.F.);
#26441=ADVANCED_FACE('',(#3628),#2407,.T.);
#26442=ADVANCED_FACE('',(#3629),#2408,.F.);
#26443=ADVANCED_FACE('',(#3630),#2409,.T.);
#26444=ADVANCED_FACE('',(#3631),#2410,.F.);
#26445=ADVANCED_FACE('',(#3632),#2411,.T.);
#26446=ADVANCED_FACE('',(#3633),#2412,.F.);
#26447=ADVANCED_FACE('',(#3634),#2413,.T.);
#26448=ADVANCED_FACE('',(#3635),#2414,.T.);
#26449=ADVANCED_FACE('',(#3636),#2415,.F.);
#26450=ADVANCED_FACE('',(#3637),#2416,.F.);
#26451=ADVANCED_FACE('',(#3638),#2417,.T.);
#26452=ADVANCED_FACE('',(#3639),#2418,.T.);
#26453=ADVANCED_FACE('',(#3640),#2419,.F.);
#26454=ADVANCED_FACE('',(#3641),#2420,.F.);
#26455=ADVANCED_FACE('',(#3642),#2421,.T.);
#26456=ADVANCED_FACE('',(#3643),#2422,.T.);
#26457=ADVANCED_FACE('',(#3644),#2423,.F.);
#26458=ADVANCED_FACE('',(#3645),#738,.F.);
#26459=ADVANCED_FACE('',(#3646,#878),#2424,.F.);
#26460=ADVANCED_FACE('',(#3647),#739,.F.);
#26461=ADVANCED_FACE('',(#3648),#25347,.F.);
#26462=ADVANCED_FACE('',(#3649,#879),#2425,.T.);
#26463=ADVANCED_FACE('',(#3650),#25348,.T.);
#26464=ADVANCED_FACE('',(#3651,#880,#881,#882,#883,#884,#885,#886),#740,
 .T.);
#26465=ADVANCED_FACE('',(#3652),#135,.T.);
#26884=CLOSED_SHELL('',(#26418,#26419,#26420,#26421,#26422,#26423,#26424,
#26425,#26426,#26427,#26428,#26429,#26430,#26431,#26432,#26433,#26434,#26435,
#26436,#26437,#26438,#26439,#26440,#26441,#26442,#26443,#26444,#26445,#26446,
#26447,#26448,#26449,#26450,#26451,#26452,#26453,#26454,#26455,#26456,#26457,
#26458,#26459,#26460,#26461,#26462,#26463,#26464,#26465));
#28305=AXIS2_PLACEMENT_3D('',#63694,#33402,#33403);
#28306=AXIS2_PLACEMENT_3D('',#63695,#33404,#33405);
#28307=AXIS2_PLACEMENT_3D('',#63704,#33410,#33411);
#28308=AXIS2_PLACEMENT_3D('',#63706,#33412,#33413);
#28309=AXIS2_PLACEMENT_3D('',#63709,#33415,#33416);
#28310=AXIS2_PLACEMENT_3D('',#63710,#33417,#33418);
#28311=AXIS2_PLACEMENT_3D('',#63716,#33422,#33423);
#28312=AXIS2_PLACEMENT_3D('',#63725,#33428,#33429);
#28313=AXIS2_PLACEMENT_3D('',#63727,#33430,#33431);
#28314=AXIS2_PLACEMENT_3D('',#63730,#33433,#33434);
#28315=AXIS2_PLACEMENT_3D('',#63731,#33435,#33436);
#28316=AXIS2_PLACEMENT_3D('',#63737,#33440,#33441);
#28317=AXIS2_PLACEMENT_3D('',#63746,#33446,#33447);
#28318=AXIS2_PLACEMENT_3D('',#63748,#33448,#33449);
#28319=AXIS2_PLACEMENT_3D('',#63751,#33451,#33452);
#28320=AXIS2_PLACEMENT_3D('',#63752,#33453,#33454);
#28321=AXIS2_PLACEMENT_3D('',#63758,#33458,#33459);
#28322=AXIS2_PLACEMENT_3D('',#63767,#33464,#33465);
#28323=AXIS2_PLACEMENT_3D('',#63769,#33466,#33467);
#28324=AXIS2_PLACEMENT_3D('',#63772,#33469,#33470);
#28325=AXIS2_PLACEMENT_3D('',#63773,#33471,#33472);
#28326=AXIS2_PLACEMENT_3D('',#63779,#33476,#33477);
#28327=AXIS2_PLACEMENT_3D('',#63788,#33482,#33483);
#28328=AXIS2_PLACEMENT_3D('',#63790,#33484,#33485);
#28329=AXIS2_PLACEMENT_3D('',#63793,#33487,#33488);
#28330=AXIS2_PLACEMENT_3D('',#63794,#33489,#33490);
#28331=AXIS2_PLACEMENT_3D('',#63800,#33494,#33495);
#28332=AXIS2_PLACEMENT_3D('',#63809,#33500,#33501);
#28333=AXIS2_PLACEMENT_3D('',#63811,#33502,#33503);
#28334=AXIS2_PLACEMENT_3D('',#63814,#33505,#33506);
#28335=AXIS2_PLACEMENT_3D('',#63815,#33507,#33508);
#28336=AXIS2_PLACEMENT_3D('',#63821,#33512,#33513);
#28337=AXIS2_PLACEMENT_3D('',#63830,#33518,#33519);
#28338=AXIS2_PLACEMENT_3D('',#63832,#33520,#33521);
#28339=AXIS2_PLACEMENT_3D('',#63835,#33523,#33524);
#28340=AXIS2_PLACEMENT_3D('',#63836,#33525,#33526);
#28341=AXIS2_PLACEMENT_3D('',#63842,#33530,#33531);
#28342=AXIS2_PLACEMENT_3D('',#63851,#33536,#33537);
#28343=AXIS2_PLACEMENT_3D('',#63853,#33538,#33539);
#28344=AXIS2_PLACEMENT_3D('',#63856,#33541,#33542);
#28345=AXIS2_PLACEMENT_3D('',#63857,#33543,#33544);
#28346=AXIS2_PLACEMENT_3D('',#63863,#33548,#33549);
#28347=AXIS2_PLACEMENT_3D('',#63864,#33550,#33551);
#28348=AXIS2_PLACEMENT_3D('',#63865,#33552,#33553);
#28349=AXIS2_PLACEMENT_3D('',#63866,#33554,#33555);
#28350=AXIS2_PLACEMENT_3D('',#63867,#33556,#33557);
#28351=AXIS2_PLACEMENT_3D('',#63869,#33558,#33559);
#28352=AXIS2_PLACEMENT_3D('',#63870,#33560,#33561);
#28353=AXIS2_PLACEMENT_3D('',#63871,#33562,#33563);
#28354=AXIS2_PLACEMENT_3D('',#63873,#33564,#33565);
#28355=AXIS2_PLACEMENT_3D('',#63874,#33566,#33567);
#28356=AXIS2_PLACEMENT_3D('',#63875,#33568,#33569);
#28357=AXIS2_PLACEMENT_3D('',#63876,#33570,#33571);
#28358=AXIS2_PLACEMENT_3D('',#63877,#33572,#33573);
#28359=AXIS2_PLACEMENT_3D('',#63878,#33574,#33575);
#28360=AXIS2_PLACEMENT_3D('',#63879,#33576,#33577);
#28361=AXIS2_PLACEMENT_3D('',#63880,#33578,#33579);
#28362=AXIS2_PLACEMENT_3D('',#63881,#33580,#33581);
#28363=AXIS2_PLACEMENT_3D('',#63882,#33582,#33583);
#28364=AXIS2_PLACEMENT_3D('',#63883,#33584,#33585);
#28365=AXIS2_PLACEMENT_3D('',#63884,#33586,#33587);
#28366=AXIS2_PLACEMENT_3D('',#63885,#33588,#33589);
#28367=AXIS2_PLACEMENT_3D('',#63886,#33590,#33591);
#28368=AXIS2_PLACEMENT_3D('',#63887,#33592,#33593);
#28369=AXIS2_PLACEMENT_3D('',#63888,#33594,#33595);
#28370=AXIS2_PLACEMENT_3D('',#63889,#33596,#33597);
#28371=AXIS2_PLACEMENT_3D('',#63890,#33598,#33599);
#28372=AXIS2_PLACEMENT_3D('',#63891,#33600,#33601);
#28373=AXIS2_PLACEMENT_3D('',#63892,#33602,#33603);
#28374=AXIS2_PLACEMENT_3D('',#63893,#33604,#33605);
#28375=AXIS2_PLACEMENT_3D('',#63894,#33606,#33607);
#28376=AXIS2_PLACEMENT_3D('',#63895,#33608,#33609);
#28377=AXIS2_PLACEMENT_3D('',#63896,#33610,#33611);
#28378=AXIS2_PLACEMENT_3D('',#63897,#33612,#33613);
#28379=AXIS2_PLACEMENT_3D('',#63898,#33614,#33615);
#28380=AXIS2_PLACEMENT_3D('',#63899,#33616,#33617);
#28381=AXIS2_PLACEMENT_3D('',#63901,#33618,#33619);
#28382=AXIS2_PLACEMENT_3D('',#63904,#33621,#33622);
#28383=AXIS2_PLACEMENT_3D('',#63905,#33623,#33624);
#28384=AXIS2_PLACEMENT_3D('',#63907,#33625,#33626);
#28385=AXIS2_PLACEMENT_3D('',#63908,#33627,#33628);
#28386=AXIS2_PLACEMENT_3D('',#63911,#33630,#33631);
#28387=AXIS2_PLACEMENT_3D('',#63912,#33632,#33633);
#28388=AXIS2_PLACEMENT_3D('',#63915,#33635,#33636);
#28389=AXIS2_PLACEMENT_3D('',#63917,#33637,#33638);
#28390=AXIS2_PLACEMENT_3D('',#63918,#33639,#33640);
#28391=AXIS2_PLACEMENT_3D('',#63920,#33641,#33642);
#28392=AXIS2_PLACEMENT_3D('',#63922,#33644,#33645);
#28393=AXIS2_PLACEMENT_3D('',#63924,#33646,#33647);
#28394=AXIS2_PLACEMENT_3D('',#63927,#33650,#33651);
#28395=AXIS2_PLACEMENT_3D('',#63929,#33652,#33653);
#33402=DIRECTION('axis',(0.,0.,1.));
#33403=DIRECTION('refdir',(1.,0.,0.));
#33404=DIRECTION('center_axis',(0.942522113366887,-0.334143780152224,0.));
#33405=DIRECTION('ref_axis',(0.,0.,-1.));
#33406=DIRECTION('',(-0.334143780152224,-0.942522113366887,0.));
#33407=DIRECTION('',(0.,0.,1.));
#33408=DIRECTION('',(0.334143780152224,0.942522113366887,0.));
#33409=DIRECTION('',(0.,0.,-1.));
#33410=DIRECTION('center_axis',(0.,0.,1.));
#33411=DIRECTION('ref_axis',(1.,0.,0.));
#33412=DIRECTION('center_axis',(0.,0.,1.));
#33413=DIRECTION('ref_axis',(1.,0.,0.));
#33414=DIRECTION('',(0.,0.,-1.));
#33415=DIRECTION('center_axis',(0.,0.,1.));
#33416=DIRECTION('ref_axis',(1.,0.,0.));
#33417=DIRECTION('center_axis',(0.334143780152225,-0.942522113366886,0.));
#33418=DIRECTION('ref_axis',(0.,0.,-1.));
#33419=DIRECTION('',(0.942522113366886,0.334143780152225,0.));
#33420=DIRECTION('',(-0.942522113366886,-0.334143780152225,0.));
#33421=DIRECTION('',(0.,0.,1.));
#33422=DIRECTION('center_axis',(-0.942522113366889,-0.334143780152217,0.));
#33423=DIRECTION('ref_axis',(0.,0.,1.));
#33424=DIRECTION('',(0.334143780152217,-0.942522113366889,0.));
#33425=DIRECTION('',(0.,0.,-1.));
#33426=DIRECTION('',(-0.334143780152217,0.942522113366889,0.));
#33427=DIRECTION('',(0.,0.,1.));
#33428=DIRECTION('center_axis',(0.,0.,1.));
#33429=DIRECTION('ref_axis',(1.,0.,0.));
#33430=DIRECTION('center_axis',(0.,0.,1.));
#33431=DIRECTION('ref_axis',(1.,0.,0.));
#33432=DIRECTION('',(0.,0.,1.));
#33433=DIRECTION('center_axis',(0.,0.,1.));
#33434=DIRECTION('ref_axis',(1.,0.,0.));
#33435=DIRECTION('center_axis',(-0.334143780152224,-0.942522113366887,0.));
#33436=DIRECTION('ref_axis',(0.,0.,-1.));
#33437=DIRECTION('',(-0.942522113366887,0.334143780152224,0.));
#33438=DIRECTION('',(0.942522113366887,-0.334143780152224,0.));
#33439=DIRECTION('',(0.,0.,-1.));
#33440=DIRECTION('center_axis',(0.902739110616947,0.430188444943055,0.));
#33441=DIRECTION('ref_axis',(0.,0.,-1.));
#33442=DIRECTION('',(0.430188444943055,-0.902739110616947,0.));
#33443=DIRECTION('',(0.,0.,1.));
#33444=DIRECTION('',(-0.430188444943055,0.902739110616947,0.));
#33445=DIRECTION('',(0.,0.,-1.));
#33446=DIRECTION('center_axis',(0.,0.,1.));
#33447=DIRECTION('ref_axis',(-1.,-1.22464679914735E-16,0.));
#33448=DIRECTION('center_axis',(0.,0.,1.));
#33449=DIRECTION('ref_axis',(1.,0.,0.));
#33450=DIRECTION('',(0.,0.,-1.));
#33451=DIRECTION('center_axis',(0.,0.,1.));
#33452=DIRECTION('ref_axis',(1.,0.,0.));
#33453=DIRECTION('center_axis',(0.902739110616947,-0.430188444943055,0.));
#33454=DIRECTION('ref_axis',(0.,0.,-1.));
#33455=DIRECTION('',(0.430188444943055,0.902739110616947,0.));
#33456=DIRECTION('',(-0.430188444943055,-0.902739110616947,0.));
#33457=DIRECTION('',(0.,0.,1.));
#33458=DIRECTION('center_axis',(0.430188444943055,0.902739110616947,0.));
#33459=DIRECTION('ref_axis',(0.,0.,1.));
#33460=DIRECTION('',(-0.902739110616947,0.430188444943055,0.));
#33461=DIRECTION('',(0.,0.,-1.));
#33462=DIRECTION('',(0.902739110616947,-0.430188444943055,0.));
#33463=DIRECTION('',(0.,0.,1.));
#33464=DIRECTION('center_axis',(0.,0.,1.));
#33465=DIRECTION('ref_axis',(1.,0.,0.));
#33466=DIRECTION('center_axis',(0.,0.,1.));
#33467=DIRECTION('ref_axis',(1.,0.,0.));
#33468=DIRECTION('',(0.,0.,1.));
#33469=DIRECTION('center_axis',(0.,0.,1.));
#33470=DIRECTION('ref_axis',(1.,0.,0.));
#33471=DIRECTION('center_axis',(-0.430188444943055,0.902739110616947,0.));
#33472=DIRECTION('ref_axis',(0.,0.,1.));
#33473=DIRECTION('',(0.902739110616947,0.430188444943055,0.));
#33474=DIRECTION('',(-0.902739110616947,-0.430188444943055,0.));
#33475=DIRECTION('',(0.,0.,-1.));
#33476=DIRECTION('center_axis',(0.334143780152223,0.942522113366887,0.));
#33477=DIRECTION('ref_axis',(0.,0.,1.));
#33478=DIRECTION('',(0.942522113366887,-0.334143780152223,0.));
#33479=DIRECTION('',(0.,0.,1.));
#33480=DIRECTION('',(-0.942522113366887,0.334143780152223,0.));
#33481=DIRECTION('',(0.,0.,-1.));
#33482=DIRECTION('center_axis',(0.,0.,1.));
#33483=DIRECTION('ref_axis',(1.,0.,0.));
#33484=DIRECTION('center_axis',(0.,0.,1.));
#33485=DIRECTION('ref_axis',(1.,0.,0.));
#33486=DIRECTION('',(0.,0.,-1.));
#33487=DIRECTION('center_axis',(0.,0.,1.));
#33488=DIRECTION('ref_axis',(1.,0.,0.));
#33489=DIRECTION('center_axis',(0.942522113366887,0.334143780152223,0.));
#33490=DIRECTION('ref_axis',(0.,0.,-1.));
#33491=DIRECTION('',(-0.334143780152223,0.942522113366887,0.));
#33492=DIRECTION('',(0.334143780152223,-0.942522113366887,0.));
#33493=DIRECTION('',(0.,0.,1.));
#33494=DIRECTION('center_axis',(-0.334143780152223,0.942522113366887,0.));
#33495=DIRECTION('ref_axis',(0.,0.,1.));
#33496=DIRECTION('',(-0.942522113366887,-0.334143780152223,0.));
#33497=DIRECTION('',(0.,0.,-1.));
#33498=DIRECTION('',(0.942522113366887,0.334143780152223,0.));
#33499=DIRECTION('',(0.,0.,1.));
#33500=DIRECTION('center_axis',(0.,0.,1.));
#33501=DIRECTION('ref_axis',(1.,0.,0.));
#33502=DIRECTION('center_axis',(0.,0.,1.));
#33503=DIRECTION('ref_axis',(1.,0.,0.));
#33504=DIRECTION('',(0.,0.,1.));
#33505=DIRECTION('center_axis',(0.,0.,1.));
#33506=DIRECTION('ref_axis',(1.,0.,0.));
#33507=DIRECTION('center_axis',(-0.942522113366887,0.334143780152223,0.));
#33508=DIRECTION('ref_axis',(0.,0.,1.));
#33509=DIRECTION('',(0.334143780152223,0.942522113366887,0.));
#33510=DIRECTION('',(-0.334143780152223,-0.942522113366887,0.));
#33511=DIRECTION('',(0.,0.,-1.));
#33512=DIRECTION('center_axis',(-0.902739110616947,0.430188444943055,0.));
#33513=DIRECTION('ref_axis',(0.,0.,1.));
#33514=DIRECTION('',(-0.430188444943055,-0.902739110616947,0.));
#33515=DIRECTION('',(0.,0.,-1.));
#33516=DIRECTION('',(0.430188444943055,0.902739110616947,0.));
#33517=DIRECTION('',(0.,0.,1.));
#33518=DIRECTION('center_axis',(0.,0.,1.));
#33519=DIRECTION('ref_axis',(1.,0.,0.));
#33520=DIRECTION('center_axis',(0.,0.,1.));
#33521=DIRECTION('ref_axis',(1.,0.,0.));
#33522=DIRECTION('',(0.,0.,1.));
#33523=DIRECTION('center_axis',(0.,0.,1.));
#33524=DIRECTION('ref_axis',(1.,0.,0.));
#33525=DIRECTION('center_axis',(-0.902739110616947,-0.430188444943055,0.));
#33526=DIRECTION('ref_axis',(0.,0.,1.));
#33527=DIRECTION('',(-0.430188444943055,0.902739110616947,0.));
#33528=DIRECTION('',(0.430188444943055,-0.902739110616947,0.));
#33529=DIRECTION('',(0.,0.,-1.));
#33530=DIRECTION('center_axis',(-0.430188444943055,-0.902739110616947,0.));
#33531=DIRECTION('ref_axis',(0.,0.,-1.));
#33532=DIRECTION('',(0.902739110616947,-0.430188444943055,0.));
#33533=DIRECTION('',(0.,0.,-1.));
#33534=DIRECTION('',(-0.902739110616947,0.430188444943055,0.));
#33535=DIRECTION('',(0.,0.,1.));
#33536=DIRECTION('center_axis',(0.,0.,1.));
#33537=DIRECTION('ref_axis',(1.,0.,0.));
#33538=DIRECTION('center_axis',(0.,0.,1.));
#33539=DIRECTION('ref_axis',(1.,0.,0.));
#33540=DIRECTION('',(0.,0.,1.));
#33541=DIRECTION('center_axis',(0.,0.,1.));
#33542=DIRECTION('ref_axis',(1.,0.,0.));
#33543=DIRECTION('center_axis',(0.430188444943055,-0.902739110616947,0.));
#33544=DIRECTION('ref_axis',(0.,0.,-1.));
#33545=DIRECTION('',(-0.902739110616947,-0.430188444943055,0.));
#33546=DIRECTION('',(0.902739110616947,0.430188444943055,0.));
#33547=DIRECTION('',(0.,0.,-1.));
#33548=DIRECTION('center_axis',(0.,0.,1.));
#33549=DIRECTION('ref_axis',(1.,0.,0.));
#33550=DIRECTION('center_axis',(0.,0.,1.));
#33551=DIRECTION('ref_axis',(1.,0.,0.));
#33552=DIRECTION('center_axis',(0.,0.,1.));
#33553=DIRECTION('ref_axis',(1.,0.,0.));
#33554=DIRECTION('center_axis',(0.,0.,-1.));
#33555=DIRECTION('ref_axis',(1.,0.,0.));
#33556=DIRECTION('center_axis',(0.,0.,1.));
#33557=DIRECTION('ref_axis',(1.,0.,0.));
#33558=DIRECTION('center_axis',(0.,0.,1.));
#33559=DIRECTION('ref_axis',(1.,0.,0.));
#33560=DIRECTION('center_axis',(0.,0.,1.));
#33561=DIRECTION('ref_axis',(1.,0.,0.));
#33562=DIRECTION('center_axis',(0.,0.,1.));
#33563=DIRECTION('ref_axis',(1.,0.,0.));
#33564=DIRECTION('center_axis',(0.,0.,-1.));
#33565=DIRECTION('ref_axis',(1.,0.,0.));
#33566=DIRECTION('center_axis',(0.,0.,-1.));
#33567=DIRECTION('ref_axis',(1.,0.,0.));
#33568=DIRECTION('center_axis',(0.,0.,1.));
#33569=DIRECTION('ref_axis',(1.,0.,0.));
#33570=DIRECTION('center_axis',(0.,0.,1.));
#33571=DIRECTION('ref_axis',(1.,0.,0.));
#33572=DIRECTION('center_axis',(0.,0.,1.));
#33573=DIRECTION('ref_axis',(1.,0.,0.));
#33574=DIRECTION('center_axis',(0.,0.,-1.));
#33575=DIRECTION('ref_axis',(1.,0.,0.));
#33576=DIRECTION('center_axis',(0.,0.,1.));
#33577=DIRECTION('ref_axis',(1.,0.,0.));
#33578=DIRECTION('center_axis',(0.,0.,-1.));
#33579=DIRECTION('ref_axis',(1.,0.,0.));
#33580=DIRECTION('center_axis',(0.,0.,1.));
#33581=DIRECTION('ref_axis',(1.,0.,0.));
#33582=DIRECTION('center_axis',(0.,0.,1.));
#33583=DIRECTION('ref_axis',(1.,0.,0.));
#33584=DIRECTION('center_axis',(0.,0.,1.));
#33585=DIRECTION('ref_axis',(1.,0.,0.));
#33586=DIRECTION('center_axis',(0.,0.,1.));
#33587=DIRECTION('ref_axis',(1.,0.,0.));
#33588=DIRECTION('center_axis',(0.,0.,1.));
#33589=DIRECTION('ref_axis',(1.,0.,0.));
#33590=DIRECTION('center_axis',(0.,0.,-1.));
#33591=DIRECTION('ref_axis',(1.,0.,0.));
#33592=DIRECTION('center_axis',(0.,0.,1.));
#33593=DIRECTION('ref_axis',(1.,0.,0.));
#33594=DIRECTION('center_axis',(0.,0.,-1.));
#33595=DIRECTION('ref_axis',(1.,0.,0.));
#33596=DIRECTION('center_axis',(0.,0.,1.));
#33597=DIRECTION('ref_axis',(1.,0.,0.));
#33598=DIRECTION('center_axis',(0.,0.,1.));
#33599=DIRECTION('ref_axis',(1.,0.,0.));
#33600=DIRECTION('center_axis',(0.,0.,1.));
#33601=DIRECTION('ref_axis',(1.,0.,0.));
#33602=DIRECTION('center_axis',(0.,0.,1.));
#33603=DIRECTION('ref_axis',(1.,0.,0.));
#33604=DIRECTION('center_axis',(0.,0.,1.));
#33605=DIRECTION('ref_axis',(1.,0.,0.));
#33606=DIRECTION('center_axis',(0.,0.,-1.));
#33607=DIRECTION('ref_axis',(1.,0.,0.));
#33608=DIRECTION('center_axis',(0.,0.,1.));
#33609=DIRECTION('ref_axis',(1.,0.,0.));
#33610=DIRECTION('center_axis',(0.,0.,-1.));
#33611=DIRECTION('ref_axis',(1.,0.,0.));
#33612=DIRECTION('center_axis',(0.,0.,1.));
#33613=DIRECTION('ref_axis',(1.,0.,0.));
#33614=DIRECTION('center_axis',(0.,0.,1.));
#33615=DIRECTION('ref_axis',(1.,0.,0.));
#33616=DIRECTION('center_axis',(0.,0.,1.));
#33617=DIRECTION('ref_axis',(1.,0.,0.));
#33618=DIRECTION('center_axis',(0.,0.,1.));
#33619=DIRECTION('ref_axis',(1.,0.,0.));
#33620=DIRECTION('',(0.,0.,1.));
#33621=DIRECTION('center_axis',(0.,0.,1.));
#33622=DIRECTION('ref_axis',(1.,0.,0.));
#33623=DIRECTION('center_axis',(0.,0.,1.));
#33624=DIRECTION('ref_axis',(1.,0.,0.));
#33625=DIRECTION('center_axis',(0.,0.,1.));
#33626=DIRECTION('ref_axis',(1.,0.,0.));
#33627=DIRECTION('center_axis',(0.,0.,1.));
#33628=DIRECTION('ref_axis',(1.,0.,0.));
#33629=DIRECTION('',(0.,0.,1.));
#33630=DIRECTION('center_axis',(0.,0.,1.));
#33631=DIRECTION('ref_axis',(1.,0.,0.));
#33632=DIRECTION('center_axis',(0.,0.,-1.));
#33633=DIRECTION('ref_axis',(1.,0.,0.));
#33634=DIRECTION('',(0.857167300702114,1.04972719113862E-16,0.515038074910052));
#33635=DIRECTION('center_axis',(0.,0.,-1.));
#33636=DIRECTION('ref_axis',(-1.,0.,0.));
#33637=DIRECTION('center_axis',(0.,0.,1.));
#33638=DIRECTION('ref_axis',(1.,0.,0.));
#33639=DIRECTION('center_axis',(0.,0.,1.));
#33640=DIRECTION('ref_axis',(1.,0.,0.));
#33641=DIRECTION('center_axis',(0.,0.,1.));
#33642=DIRECTION('ref_axis',(1.,0.,0.));
#33643=DIRECTION('',(0.707106781186543,8.65956056235488E-17,-0.707106781186552));
#33644=DIRECTION('center_axis',(0.,0.,1.));
#33645=DIRECTION('ref_axis',(1.,0.,0.));
#33646=DIRECTION('center_axis',(0.,0.,1.));
#33647=DIRECTION('ref_axis',(1.,0.,0.));
#33648=DIRECTION('',(0.,0.,-1.));
#33649=DIRECTION('',(0.,0.,-1.));
#33650=DIRECTION('center_axis',(6.12323399573677E-17,0.,1.));
#33651=DIRECTION('ref_axis',(1.,0.,0.));
#33652=DIRECTION('center_axis',(1.22464679914735E-16,-1.,0.));
#33653=DIRECTION('ref_axis',(-1.,-1.22464679914735E-16,0.));
#63694=CARTESIAN_POINT('',(0.,0.,0.));
#63695=CARTESIAN_POINT('Origin',(1.51164990307781,-1.90362339303322,56.979171306613));
#63696=CARTESIAN_POINT('',(1.46950013062437,-2.02251560342435,56.6));
#63697=CARTESIAN_POINT('',(1.55379967553124,-1.78473118264209,56.6));
#63698=CARTESIAN_POINT('',(1.54374745319659,-1.81308556899211,56.6));
#63699=CARTESIAN_POINT('',(1.55379967553124,-1.78473118264209,57.55834261));
#63700=CARTESIAN_POINT('',(1.55379967553124,-1.78473118264209,56.979171306613));
#63701=CARTESIAN_POINT('',(1.46950013062437,-2.02251560342435,57.55834261));
#63702=CARTESIAN_POINT('',(1.54374745319659,-1.81308556899211,57.55834261));
#63703=CARTESIAN_POINT('',(1.46950013062437,-2.02251560342435,56.979171306613));
#63704=CARTESIAN_POINT('Origin',(1.8031222920257,-1.8031222920257,56.6));
#63705=CARTESIAN_POINT('',(1.78473118264209,-1.55379967553124,56.6));
#63706=CARTESIAN_POINT('Origin',(1.8031222920257,-1.8031222920257,56.6));
#63707=CARTESIAN_POINT('',(1.78473118264209,-1.55379967553124,57.55834261));
#63708=CARTESIAN_POINT('',(1.78473118264209,-1.55379967553124,56.979171306613));
#63709=CARTESIAN_POINT('Origin',(1.8031222920257,-1.8031222920257,57.55834261));
#63710=CARTESIAN_POINT('Origin',(1.90362339303322,-1.51164990307781,56.979171306613));
#63711=CARTESIAN_POINT('',(2.02251560342435,-1.46950013062437,57.55834261));
#63712=CARTESIAN_POINT('',(1.81308556899211,-1.54374745319659,57.55834261));
#63713=CARTESIAN_POINT('',(2.02251560342435,-1.46950013062437,56.6));
#63714=CARTESIAN_POINT('',(1.81308556899211,-1.54374745319659,56.6));
#63715=CARTESIAN_POINT('',(2.02251560342435,-1.46950013062437,56.979171306613));
#63716=CARTESIAN_POINT('Origin',(-1.51164990307781,-1.90362339303322,56.979171306613));
#63717=CARTESIAN_POINT('',(-1.46950013062437,-2.02251560342435,57.55834261));
#63718=CARTESIAN_POINT('',(-1.55379967553124,-1.78473118264209,57.55834261));
#63719=CARTESIAN_POINT('',(-1.54374745319659,-1.81308556899211,57.55834261));
#63720=CARTESIAN_POINT('',(-1.55379967553124,-1.78473118264209,56.6));
#63721=CARTESIAN_POINT('',(-1.55379967553124,-1.78473118264209,56.979171306613));
#63722=CARTESIAN_POINT('',(-1.46950013062437,-2.02251560342435,56.6));
#63723=CARTESIAN_POINT('',(-1.54374745319659,-1.81308556899211,56.6));
#63724=CARTESIAN_POINT('',(-1.46950013062437,-2.02251560342435,56.979171306613));
#63725=CARTESIAN_POINT('Origin',(-1.8031222920257,-1.8031222920257,56.6));
#63726=CARTESIAN_POINT('',(-1.78473118264209,-1.55379967553124,57.55834261));
#63727=CARTESIAN_POINT('Origin',(-1.8031222920257,-1.8031222920257,57.55834261));
#63728=CARTESIAN_POINT('',(-1.78473118264209,-1.55379967553124,56.6));
#63729=CARTESIAN_POINT('',(-1.78473118264209,-1.55379967553124,56.979171306613));
#63730=CARTESIAN_POINT('Origin',(-1.8031222920257,-1.8031222920257,56.6));
#63731=CARTESIAN_POINT('Origin',(-1.90362339303322,-1.51164990307781,56.979171306613));
#63732=CARTESIAN_POINT('',(-2.02251560342435,-1.46950013062437,56.6));
#63733=CARTESIAN_POINT('',(-1.81308556899211,-1.54374745319659,56.6));
#63734=CARTESIAN_POINT('',(-2.02251560342435,-1.46950013062437,57.55834261));
#63735=CARTESIAN_POINT('',(-1.81308556899211,-1.54374745319659,57.55834261));
#63736=CARTESIAN_POINT('',(-2.02251560342435,-1.46950013062437,56.979171306613));
#63737=CARTESIAN_POINT('Origin',(2.41496290728544,-0.277167112792829,56.979171306613));
#63738=CARTESIAN_POINT('',(2.46922800555597,-0.391040990917948,56.6));
#63739=CARTESIAN_POINT('',(2.36069780901491,-0.16329323466771,56.6));
#63740=CARTESIAN_POINT('',(2.37363939330056,-0.190450808111023,56.6));
#63741=CARTESIAN_POINT('',(2.36069780901491,-0.16329323466771,57.55834261));
#63742=CARTESIAN_POINT('',(2.36069780901491,-0.16329323466771,56.979171306613));
#63743=CARTESIAN_POINT('',(2.46922800555597,-0.391040990917948,57.55834261));
#63744=CARTESIAN_POINT('',(2.37363939330056,-0.190450808111023,57.55834261));
#63745=CARTESIAN_POINT('',(2.46922800555597,-0.391040990917948,56.979171306613));
#63746=CARTESIAN_POINT('Origin',(2.55,0.,56.6));
#63747=CARTESIAN_POINT('',(2.36069780901491,0.16329323466771,56.6));
#63748=CARTESIAN_POINT('Origin',(2.55,0.,56.6));
#63749=CARTESIAN_POINT('',(2.36069780901491,0.16329323466771,57.55834261));
#63750=CARTESIAN_POINT('',(2.36069780901491,0.16329323466771,56.979171306613));
#63751=CARTESIAN_POINT('Origin',(2.55,0.,57.55834261));
#63752=CARTESIAN_POINT('Origin',(2.41496290728544,0.277167112792829,56.979171306613));
#63753=CARTESIAN_POINT('',(2.46922800555597,0.391040990917948,57.55834261));
#63754=CARTESIAN_POINT('',(2.37363939330056,0.190450808111023,57.55834261));
#63755=CARTESIAN_POINT('',(2.46922800555597,0.391040990917948,56.6));
#63756=CARTESIAN_POINT('',(2.37363939330056,0.190450808111023,56.6));
#63757=CARTESIAN_POINT('',(2.46922800555597,0.391040990917948,56.979171306613));
#63758=CARTESIAN_POINT('Origin',(-0.277167112792829,2.41496290728544,56.979171306613));
#63759=CARTESIAN_POINT('',(-0.391040990917948,2.46922800555597,57.55834261));
#63760=CARTESIAN_POINT('',(-0.16329323466771,2.36069780901491,57.55834261));
#63761=CARTESIAN_POINT('',(-0.190450808111023,2.37363939330056,57.55834261));
#63762=CARTESIAN_POINT('',(-0.16329323466771,2.36069780901491,56.6));
#63763=CARTESIAN_POINT('',(-0.16329323466771,2.36069780901491,56.979171306613));
#63764=CARTESIAN_POINT('',(-0.391040990917948,2.46922800555597,56.6));
#63765=CARTESIAN_POINT('',(-0.190450808111023,2.37363939330056,56.6));
#63766=CARTESIAN_POINT('',(-0.391040990917948,2.46922800555597,56.979171306613));
#63767=CARTESIAN_POINT('Origin',(1.56142466891288E-16,2.55,56.6));
#63768=CARTESIAN_POINT('',(0.163293234667711,2.36069780901491,57.55834261));
#63769=CARTESIAN_POINT('Origin',(1.56142466891288E-16,2.55,57.55834261));
#63770=CARTESIAN_POINT('',(0.163293234667711,2.36069780901491,56.6));
#63771=CARTESIAN_POINT('',(0.163293234667711,2.36069780901491,56.979171306613));
#63772=CARTESIAN_POINT('Origin',(1.56142466891288E-16,2.55,56.6));
#63773=CARTESIAN_POINT('Origin',(0.277167112792829,2.41496290728544,56.979171306613));
#63774=CARTESIAN_POINT('',(0.391040990917948,2.46922800555597,56.6));
#63775=CARTESIAN_POINT('',(0.190450808111023,2.37363939330056,56.6));
#63776=CARTESIAN_POINT('',(0.391040990917948,2.46922800555597,57.55834261));
#63777=CARTESIAN_POINT('',(0.190450808111023,2.37363939330056,57.55834261));
#63778=CARTESIAN_POINT('',(0.391040990917948,2.46922800555597,56.979171306613));
#63779=CARTESIAN_POINT('Origin',(1.90362339303322,1.51164990307781,56.979171306613));
#63780=CARTESIAN_POINT('',(2.02251560342435,1.46950013062437,56.6));
#63781=CARTESIAN_POINT('',(1.78473118264209,1.55379967553124,56.6));
#63782=CARTESIAN_POINT('',(1.81308556899211,1.54374745319659,56.6));
#63783=CARTESIAN_POINT('',(1.78473118264209,1.55379967553124,57.55834261));
#63784=CARTESIAN_POINT('',(1.78473118264209,1.55379967553124,56.979171306613));
#63785=CARTESIAN_POINT('',(2.02251560342435,1.46950013062437,57.55834261));
#63786=CARTESIAN_POINT('',(1.81308556899211,1.54374745319659,57.55834261));
#63787=CARTESIAN_POINT('',(2.02251560342435,1.46950013062437,56.979171306613));
#63788=CARTESIAN_POINT('Origin',(1.8031222920257,1.8031222920257,56.6));
#63789=CARTESIAN_POINT('',(1.55379967553124,1.78473118264209,56.6));
#63790=CARTESIAN_POINT('Origin',(1.8031222920257,1.8031222920257,56.6));
#63791=CARTESIAN_POINT('',(1.55379967553124,1.78473118264209,57.55834261));
#63792=CARTESIAN_POINT('',(1.55379967553124,1.78473118264209,56.979171306613));
#63793=CARTESIAN_POINT('Origin',(1.8031222920257,1.8031222920257,57.55834261));
#63794=CARTESIAN_POINT('Origin',(1.51164990307781,1.90362339303322,56.979171306613));
#63795=CARTESIAN_POINT('',(1.46950013062437,2.02251560342435,57.55834261));
#63796=CARTESIAN_POINT('',(1.54374745319659,1.81308556899211,57.55834261));
#63797=CARTESIAN_POINT('',(1.46950013062437,2.02251560342435,56.6));
#63798=CARTESIAN_POINT('',(1.54374745319659,1.81308556899211,56.6));
#63799=CARTESIAN_POINT('',(1.46950013062437,2.02251560342435,56.979171306613));
#63800=CARTESIAN_POINT('Origin',(-1.90362339303322,1.51164990307781,56.979171306613));
#63801=CARTESIAN_POINT('',(-2.02251560342435,1.46950013062437,57.55834261));
#63802=CARTESIAN_POINT('',(-1.78473118264209,1.55379967553124,57.55834261));
#63803=CARTESIAN_POINT('',(-1.81308556899211,1.54374745319659,57.55834261));
#63804=CARTESIAN_POINT('',(-1.78473118264209,1.55379967553124,56.6));
#63805=CARTESIAN_POINT('',(-1.78473118264209,1.55379967553124,56.979171306613));
#63806=CARTESIAN_POINT('',(-2.02251560342435,1.46950013062437,56.6));
#63807=CARTESIAN_POINT('',(-1.81308556899211,1.54374745319659,56.6));
#63808=CARTESIAN_POINT('',(-2.02251560342435,1.46950013062437,56.979171306613));
#63809=CARTESIAN_POINT('Origin',(-1.8031222920257,1.8031222920257,56.6));
#63810=CARTESIAN_POINT('',(-1.55379967553124,1.78473118264209,57.55834261));
#63811=CARTESIAN_POINT('Origin',(-1.8031222920257,1.8031222920257,57.55834261));
#63812=CARTESIAN_POINT('',(-1.55379967553124,1.78473118264209,56.6));
#63813=CARTESIAN_POINT('',(-1.55379967553124,1.78473118264209,56.979171306613));
#63814=CARTESIAN_POINT('Origin',(-1.8031222920257,1.8031222920257,56.6));
#63815=CARTESIAN_POINT('Origin',(-1.51164990307781,1.90362339303322,56.979171306613));
#63816=CARTESIAN_POINT('',(-1.46950013062437,2.02251560342435,56.6));
#63817=CARTESIAN_POINT('',(-1.54374745319659,1.81308556899211,56.6));
#63818=CARTESIAN_POINT('',(-1.46950013062437,2.02251560342435,57.55834261));
#63819=CARTESIAN_POINT('',(-1.54374745319659,1.81308556899211,57.55834261));
#63820=CARTESIAN_POINT('',(-1.46950013062437,2.02251560342435,56.979171306613));
#63821=CARTESIAN_POINT('Origin',(-2.41496290728544,-0.277167112792829,56.979171306613));
#63822=CARTESIAN_POINT('',(-2.46922800555597,-0.391040990917948,57.55834261));
#63823=CARTESIAN_POINT('',(-2.36069780901491,-0.16329323466771,57.55834261));
#63824=CARTESIAN_POINT('',(-2.37363939330056,-0.190450808111022,57.55834261));
#63825=CARTESIAN_POINT('',(-2.36069780901491,-0.16329323466771,56.6));
#63826=CARTESIAN_POINT('',(-2.36069780901491,-0.16329323466771,56.979171306613));
#63827=CARTESIAN_POINT('',(-2.46922800555597,-0.391040990917948,56.6));
#63828=CARTESIAN_POINT('',(-2.37363939330056,-0.190450808111022,56.6));
#63829=CARTESIAN_POINT('',(-2.46922800555597,-0.391040990917948,56.979171306613));
#63830=CARTESIAN_POINT('Origin',(-2.55,3.12284933782575E-16,56.6));
#63831=CARTESIAN_POINT('',(-2.36069780901491,0.163293234667711,57.55834261));
#63832=CARTESIAN_POINT('Origin',(-2.55,3.12284933782575E-16,57.55834261));
#63833=CARTESIAN_POINT('',(-2.36069780901491,0.163293234667711,56.6));
#63834=CARTESIAN_POINT('',(-2.36069780901491,0.163293234667711,56.979171306613));
#63835=CARTESIAN_POINT('Origin',(-2.55,3.12284933782575E-16,56.6));
#63836=CARTESIAN_POINT('Origin',(-2.41496290728544,0.27716711279283,56.979171306613));
#63837=CARTESIAN_POINT('',(-2.46922800555597,0.391040990917948,56.6));
#63838=CARTESIAN_POINT('',(-2.37363939330056,0.190450808111023,56.6));
#63839=CARTESIAN_POINT('',(-2.46922800555597,0.391040990917948,57.55834261));
#63840=CARTESIAN_POINT('',(-2.37363939330056,0.190450808111023,57.55834261));
#63841=CARTESIAN_POINT('',(-2.46922800555597,0.391040990917948,56.979171306613));
#63842=CARTESIAN_POINT('Origin',(0.277167112792829,-2.41496290728544,56.979171306613));
#63843=CARTESIAN_POINT('',(0.391040990917948,-2.46922800555597,57.55834261));
#63844=CARTESIAN_POINT('',(0.16329323466771,-2.36069780901491,57.55834261));
#63845=CARTESIAN_POINT('',(0.190450808111022,-2.37363939330056,57.55834261));
#63846=CARTESIAN_POINT('',(0.16329323466771,-2.36069780901491,56.6));
#63847=CARTESIAN_POINT('',(0.16329323466771,-2.36069780901491,56.979171306613));
#63848=CARTESIAN_POINT('',(0.391040990917948,-2.46922800555597,56.6));
#63849=CARTESIAN_POINT('',(0.190450808111022,-2.37363939330056,56.6));
#63850=CARTESIAN_POINT('',(0.391040990917948,-2.46922800555597,56.979171306613));
#63851=CARTESIAN_POINT('Origin',(-4.68427400673863E-16,-2.55,56.6));
#63852=CARTESIAN_POINT('',(-0.163293234667711,-2.36069780901491,57.55834261));
#63853=CARTESIAN_POINT('Origin',(-4.68427400673863E-16,-2.55,57.55834261));
#63854=CARTESIAN_POINT('',(-0.163293234667711,-2.36069780901491,56.6));
#63855=CARTESIAN_POINT('',(-0.163293234667711,-2.36069780901491,56.979171306613));
#63856=CARTESIAN_POINT('Origin',(-4.68427400673863E-16,-2.55,56.6));
#63857=CARTESIAN_POINT('Origin',(-0.27716711279283,-2.41496290728544,56.979171306613));
#63858=CARTESIAN_POINT('',(-0.391040990917949,-2.46922800555597,56.6));
#63859=CARTESIAN_POINT('',(-0.190450808111023,-2.37363939330056,56.6));
#63860=CARTESIAN_POINT('',(-0.391040990917949,-2.46922800555597,57.55834261));
#63861=CARTESIAN_POINT('',(-0.190450808111023,-2.37363939330056,57.55834261));
#63862=CARTESIAN_POINT('',(-0.391040990917949,-2.46922800555597,56.979171306613));
#63863=CARTESIAN_POINT('Origin',(-4.44089209850063E-16,-2.55,57.55834261));
#63864=CARTESIAN_POINT('Origin',(0.,0.,57.55834261));
#63865=CARTESIAN_POINT('Origin',(-4.44089209850063E-16,-2.55,56.6));
#63866=CARTESIAN_POINT('Origin',(0.,0.,56.6));
#63867=CARTESIAN_POINT('Origin',(-2.55,3.19189119579733E-16,57.55834261));
#63868=CARTESIAN_POINT('',(-2.5,-3.06161699786838E-16,57.55834261));
#63869=CARTESIAN_POINT('Origin',(0.,0.,57.55834261));
#63870=CARTESIAN_POINT('Origin',(0.,0.,57.55834261));
#63871=CARTESIAN_POINT('Origin',(-2.55,3.19189119579733E-16,56.6));
#63872=CARTESIAN_POINT('',(-2.5,-3.06161699786838E-16,56.6));
#63873=CARTESIAN_POINT('Origin',(0.,0.,56.6));
#63874=CARTESIAN_POINT('Origin',(0.,0.,56.6));
#63875=CARTESIAN_POINT('Origin',(-1.8031222920257,1.8031222920257,57.55834261));
#63876=CARTESIAN_POINT('Origin',(0.,0.,57.55834261));
#63877=CARTESIAN_POINT('Origin',(-1.8031222920257,1.8031222920257,56.6));
#63878=CARTESIAN_POINT('Origin',(0.,0.,56.6));
#63879=CARTESIAN_POINT('Origin',(1.8031222920257,1.8031222920257,56.6));
#63880=CARTESIAN_POINT('Origin',(0.,0.,56.6));
#63881=CARTESIAN_POINT('Origin',(1.8031222920257,1.8031222920257,57.55834261));
#63882=CARTESIAN_POINT('Origin',(0.,0.,57.55834261));
#63883=CARTESIAN_POINT('Origin',(1.66533453693773E-16,2.55,57.55834261));
#63884=CARTESIAN_POINT('Origin',(0.,0.,57.55834261));
#63885=CARTESIAN_POINT('Origin',(1.66533453693773E-16,2.55,56.6));
#63886=CARTESIAN_POINT('Origin',(0.,0.,56.6));
#63887=CARTESIAN_POINT('Origin',(2.55,0.,56.6));
#63888=CARTESIAN_POINT('Origin',(0.,0.,56.6));
#63889=CARTESIAN_POINT('Origin',(2.55,0.,57.55834261));
#63890=CARTESIAN_POINT('Origin',(0.,0.,57.55834261));
#63891=CARTESIAN_POINT('Origin',(-1.8031222920257,-1.8031222920257,57.55834261));
#63892=CARTESIAN_POINT('Origin',(0.,0.,57.55834261));
#63893=CARTESIAN_POINT('Origin',(-1.8031222920257,-1.8031222920257,56.6));
#63894=CARTESIAN_POINT('Origin',(0.,0.,56.6));
#63895=CARTESIAN_POINT('Origin',(1.8031222920257,-1.8031222920257,56.6));
#63896=CARTESIAN_POINT('Origin',(0.,0.,56.6));
#63897=CARTESIAN_POINT('Origin',(1.8031222920257,-1.8031222920257,57.55834261));
#63898=CARTESIAN_POINT('Origin',(0.,0.,57.55834261));
#63899=CARTESIAN_POINT('Origin',(0.,0.,56.035));
#63900=CARTESIAN_POINT('',(-1.3,-1.59204083889156E-16,56.));
#63901=CARTESIAN_POINT('Origin',(0.,0.,56.));
#63902=CARTESIAN_POINT('',(-1.3,-1.59204083889156E-16,56.1));
#63903=CARTESIAN_POINT('',(-1.3,-1.59204083889156E-16,56.035));
#63904=CARTESIAN_POINT('Origin',(0.,0.,56.1));
#63905=CARTESIAN_POINT('Origin',(1.205,0.,56.1));
#63906=CARTESIAN_POINT('',(-1.205,-1.47569939297256E-16,56.1));
#63907=CARTESIAN_POINT('Origin',(0.,0.,56.1));
#63908=CARTESIAN_POINT('Origin',(0.,0.,58.3));
#63909=CARTESIAN_POINT('',(-1.205,-1.47569939297256E-16,60.5));
#63910=CARTESIAN_POINT('',(-1.205,-1.47569939297256E-16,58.3));
#63911=CARTESIAN_POINT('Origin',(0.,0.,60.5));
#63912=CARTESIAN_POINT('Origin',(0.,0.,60.5));
#63913=CARTESIAN_POINT('',(0.,0.,61.2240370459282));
#63914=CARTESIAN_POINT('',(-1.205,-1.47569939297256E-16,60.5));
#63915=CARTESIAN_POINT('Origin',(2.3,0.,56.));
#63916=CARTESIAN_POINT('',(-2.3,-2.81668763803891E-16,56.));
#63917=CARTESIAN_POINT('Origin',(0.,0.,56.));
#63918=CARTESIAN_POINT('Origin',(0.,0.,56.1));
#63919=CARTESIAN_POINT('',(-2.5,-3.06161699786838E-16,56.2));
#63920=CARTESIAN_POINT('Origin',(0.,0.,56.2));
#63921=CARTESIAN_POINT('',(-2.4,-2.93915231795365E-16,56.1));
#63922=CARTESIAN_POINT('Origin',(0.,0.,56.979171306613));
#63923=CARTESIAN_POINT('',(-2.5,-3.06161699786838E-16,57.7583426132261));
#63924=CARTESIAN_POINT('Origin',(0.,0.,57.7583426132261));
#63925=CARTESIAN_POINT('',(-2.5,-3.06161699786838E-16,56.979171306613));
#63926=CARTESIAN_POINT('',(-2.5,-3.06161699786838E-16,56.979171306613));
#63927=CARTESIAN_POINT('Origin',(4.44089209850063E-16,0.,61.5));
#63928=CARTESIAN_POINT('',(1.68543680041908E-16,-3.37445951098918E-32,66.));
#63929=CARTESIAN_POINT('Origin',(4.44089209850063E-16,0.,61.5));
#70737=UNCERTAINTY_MEASURE_WITH_UNIT(LENGTH_MEASURE(0.001),#70758,
'DISTANCE_ACCURACY_VALUE',
'Maximum model space distance between geometric entities at asserted c
onnectivities');
#70740=UNCERTAINTY_MEASURE_WITH_UNIT(LENGTH_MEASURE(0.001),#70758,
'DISTANCE_ACCURACY_VALUE',
'Maximum model space distance between geometric entities at asserted c
onnectivities');
#70754=(
GEOMETRIC_REPRESENTATION_CONTEXT(3)
GLOBAL_UNCERTAINTY_ASSIGNED_CONTEXT((#70737))
GLOBAL_UNIT_ASSIGNED_CONTEXT((#70758,#70760,#70761))
REPRESENTATION_CONTEXT('','3D')
);
#70757=(
GEOMETRIC_REPRESENTATION_CONTEXT(3)
GLOBAL_UNCERTAINTY_ASSIGNED_CONTEXT((#70740))
GLOBAL_UNIT_ASSIGNED_CONTEXT((#70758,#70760,#70761))
REPRESENTATION_CONTEXT('','3D')
);
#70758=(
LENGTH_UNIT()
NAMED_UNIT(*)
SI_UNIT(.CENTI.,.METRE.)
);
#70760=(
NAMED_UNIT(*)
PLANE_ANGLE_UNIT()
SI_UNIT($,.RADIAN.)
);
#70761=(
NAMED_UNIT(*)
SI_UNIT($,.STERADIAN.)
SOLID_ANGLE_UNIT()
);
#70775=SHAPE_DEFINITION_REPRESENTATION(#70791,#70830);
#70791=PRODUCT_DEFINITION_SHAPE('',$,#70847);
#70830=SHAPE_REPRESENTATION('',(#28305),#70754);
#70833=PRODUCT_DEFINITION_CONTEXT('part definition',#70883,'design');
#70847=PRODUCT_DEFINITION('2026-10-19-02-59-02-453',
'06_Ergonomic_Ball_Knob_D90_M24',#70863,#70833);
#70863=PRODUCT_DEFINITION_FORMATION('',$,#70898);
#70883=APPLICATION_CONTEXT(
'Core Data for Automotive Mechanical Design Process');
#70884=PRODUCT_CONTEXT('part definition',#70883,'mechanical');
#70898=PRODUCT('2026-10-19-02-59-02-453',
'06_Ergonomic_Ball_Knob_D90_M24',$,(#70884));
#71034=COLOUR_RGB('Sky Blue',0.24,0.69,0.87);
#71035=FILL_AREA_STYLE_COLOUR('',#71034);
#71036=FILL_AREA_STYLE('',(#71035));
#71037=SURFACE_STYLE_FILL_AREA(#71036);
#71038=SURFACE_SIDE_STYLE('',(#71037));
#71039=SURFACE_STYLE_USAGE(.BOTH.,#71038);
#71040=PRESENTATION_STYLE_ASSIGNMENT((#71039));
ENDSEC;
END-ISO-10303-21;
